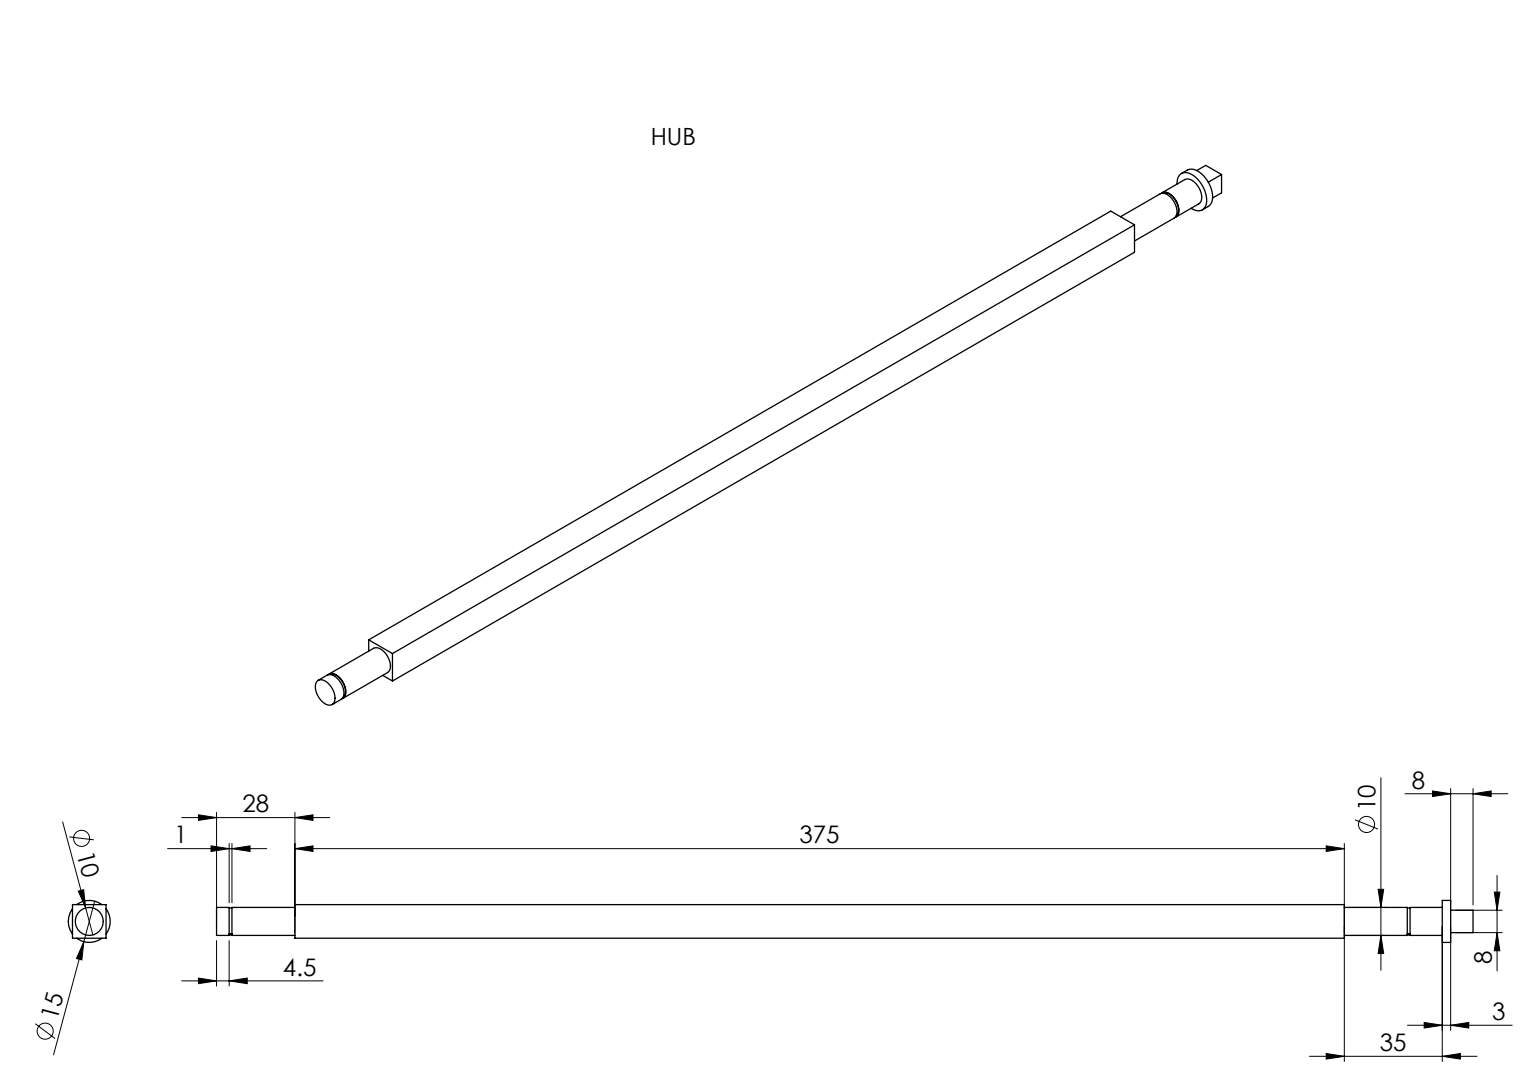
ISO-10303-21;
HEADER;
FILE_DESCRIPTION (('STEP AP214'),
    '1' );
FILE_NAME ('hub.step',
    '2026-10-27T17:01:19',
    ( '' ),
    ( '' ),
    'SwSTEP 2.0',
    'SolidWorks 2026',
    '' );
FILE_SCHEMA (( 'AUTOMOTIVE_DESIGN' ));
ENDSEC;

DATA;
#11=FACE_OUTER_BOUND ( 'NONE', #11887, .T. ) ;
#14=CARTESIAN_POINT ( 'NONE',  ( 640.0000000000000000, 160.0000000000000284, -222.5000000000000000 ) ) ;
#23=ORIENTED_EDGE ( 'NONE', *, *, #607, .T. ) ;
#30=VERTEX_POINT ( 'NONE', #596 ) ;
#33=ORIENTED_EDGE ( 'NONE', *, *, #12524, .T. ) ;
#37=CARTESIAN_POINT ( 'NONE',  ( 0.000000000000000000, 0.000000000000000000, -187.5000000000000000 ) ) ;
#38=ADVANCED_FACE ( 'NONE', ( #6155 ), #1724, .F. ) ;
#53=CARTESIAN_POINT ( 'NONE',  ( 629.0000000000000000, 166.0000000000000284, -187.5000000000000000 ) ) ;
#55=EDGE_LOOP ( 'NONE', ( #10980, #1481, #10748, #12698 ) ) ;
#70=PLANE ( 'NONE',  #7516 ) ;
#99=EDGE_LOOP ( 'NONE', ( #7071, #6114, #7487, #2779 ) ) ;
#101=DIRECTION ( 'NONE',  ( 0.000000000000000000, 0.000000000000000000, 1.000000000000000000 ) ) ;
#128=CARTESIAN_POINT ( 'NONE',  ( 630.0000000000000000, 160.0000000000000284, 215.5000000000000000 ) ) ;
#138=DIRECTION ( 'NONE',  ( -1.000000000000000000, 0.000000000000000000, 0.000000000000000000 ) ) ;
#142=CIRCLE ( 'NONE', #4214, 5.000000000000004441 ) ;
#146=DIRECTION ( 'NONE',  ( 0.000000000000000000, 0.000000000000000000, -1.000000000000000000 ) ) ;
#171=ORIENTED_EDGE ( 'NONE', *, *, #13700, .T. ) ;
#178=DIRECTION ( 'NONE',  ( 0.000000000000000000, 0.000000000000000000, -1.000000000000000000 ) ) ;
#203=AXIS2_PLACEMENT_3D ( 'NONE', #4127, #790, #8616 ) ;
#206=ADVANCED_FACE ( 'NONE', ( #6452 ), #11002, .F. ) ;
#207=ORIENTED_EDGE ( 'NONE', *, *, #12524, .F. ) ;
#218=EDGE_CURVE ( 'NONE', #4236, #7201, #9506, .T. ) ;
#230=DIRECTION ( 'NONE',  ( -1.000000000000000000, 0.000000000000000000, 0.000000000000000000 ) ) ;
#231=CARTESIAN_POINT ( 'NONE',  ( 635.0000000000000000, 160.0000000000000284, 215.5000000000000000 ) ) ;
#247=LINE ( 'NONE', #13705, #494 ) ;
#255=ORIENTED_EDGE ( 'NONE', *, *, #504, .F. ) ;
#267=CARTESIAN_POINT ( 'NONE',  ( 635.0000000000000000, 160.0000000000000284, 211.0000000000000000 ) ) ;
#274=ORIENTED_EDGE ( 'NONE', *, *, #3153, .F. ) ;
#302=EDGE_CURVE ( 'NONE', #2242, #4648, #7848, .T. ) ;
#309=EDGE_LOOP ( 'NONE', ( #11418, #2643 ) ) ;
#331=LINE ( 'NONE', #7064, #10396 ) ;
#344=VERTEX_POINT ( 'NONE', #128 ) ;
#361=DIRECTION ( 'NONE',  ( -1.000000000000000000, 0.000000000000000000, 0.000000000000000000 ) ) ;
#375=CARTESIAN_POINT ( 'NONE',  ( 637.0568832135862749, 155.4426727739092655, 210.0000000000000000 ) ) ;
#382=VECTOR ( 'NONE', #10428, 1000.000000000000000 ) ;
#383=DIRECTION ( 'NONE',  ( -2.312964634635740689E-15, 1.000000000000000000, 0.000000000000000000 ) ) ;
#390=( LENGTH_UNIT ( ) NAMED_UNIT ( * ) SI_UNIT ( .MILLI., .METRE. ) );
#403=EDGE_CURVE ( 'NONE', #12048, #8669, #5831, .T. ) ;
#426=EDGE_CURVE ( 'NONE', #4433, #3772, #8407, .T. ) ;
#433=VECTOR ( 'NONE', #6248, 1000.000000000000114 ) ;
#443=VERTEX_POINT ( 'NONE', #11657 ) ;
#471=CARTESIAN_POINT ( 'NONE',  ( 635.0000000000000000, 160.0000000000000284, -210.0000000000000000 ) ) ;
#482=( NAMED_UNIT ( * ) SI_UNIT ( $, .STERADIAN. ) SOLID_ANGLE_UNIT ( ) );
#491=VECTOR ( 'NONE', #11619, 1000.000000000000000 ) ;
#492=DIRECTION ( 'NONE',  ( 0.000000000000000000, 1.000000000000000000, 0.000000000000000000 ) ) ;
#494=VECTOR ( 'NONE', #2319, 1000.000000000000000 ) ;
#504=EDGE_CURVE ( 'NONE', #30, #10347, #1051, .T. ) ;
#509=ORIENTED_EDGE ( 'NONE', *, *, #9465, .F. ) ;
#512=VECTOR ( 'NONE', #1432, 1000.000000000000000 ) ;
#514=LINE ( 'NONE', #1705, #2365 ) ;
#515=PRODUCT_DEFINITION_FORMATION_WITH_SPECIFIED_SOURCE ( 'ANY', '', #13038, .NOT_KNOWN. ) ;
#531=EDGE_LOOP ( 'NONE', ( #7577, #12820, #549, #541 ) ) ;
#541=ORIENTED_EDGE ( 'NONE', *, *, #5828, .T. ) ;
#549=ORIENTED_EDGE ( 'NONE', *, *, #9465, .T. ) ;
#579=DIRECTION ( 'NONE',  ( -0.4113766427172328433, 0.9114654452181377708, 0.000000000000000000 ) ) ;
#587=LINE ( 'NONE', #6359, #4201 ) ;
#596=CARTESIAN_POINT ( 'NONE',  ( 630.5661054975340676, 158.1613647612965110, -210.0000000000000000 ) ) ;
#602=ORIENTED_EDGE ( 'NONE', *, *, #7925, .T. ) ;
#607=EDGE_CURVE ( 'NONE', #443, #1513, #6269, .T. ) ;
#623=AXIS2_PLACEMENT_3D ( 'NONE', #7389, #649, #7452 ) ;
#649=DIRECTION ( 'NONE',  ( 0.000000000000000000, 0.000000000000000000, 1.000000000000000000 ) ) ;
#659=DIRECTION ( 'NONE',  ( 0.9351104457158685435, 0.3543563944859322579, 0.000000000000000000 ) ) ;
#669=PLANE ( 'NONE',  #940 ) ;
#677=EDGE_CURVE ( 'NONE', #8007, #9101, #13359, .T. ) ;
#682=CARTESIAN_POINT ( 'NONE',  ( 636.7009106935324780, 155.5114698605638637, 210.0000000000000000 ) ) ;
#687=ORIENTED_EDGE ( 'NONE', *, *, #8817, .F. ) ;
#707=PLANE ( 'NONE',  #10370 ) ;
#708=VECTOR ( 'NONE', #14194, 1000.000000000000000 ) ;
#716=DIRECTION ( 'NONE',  ( 0.000000000000000000, 0.000000000000000000, -1.000000000000000000 ) ) ;
#724=ORIENTED_EDGE ( 'NONE', *, *, #11799, .T. ) ;
#728=CARTESIAN_POINT ( 'NONE',  ( 639.4338945024659324, 161.8386352387035743, 211.0000000000000000 ) ) ;
#730=DIRECTION ( 'NONE',  ( 1.000000000000000000, 0.000000000000000000, 0.000000000000000000 ) ) ;
#745=ADVANCED_FACE ( 'NONE', ( #7680 ), #12162, .T. ) ;
#771=DIRECTION ( 'NONE',  ( 1.000000000000000000, 0.000000000000000000, 0.000000000000000000 ) ) ;
#778=DIRECTION ( 'NONE',  ( -0.9237280213470676626, -0.3830490080632388272, 0.000000000000000000 ) ) ;
#790=DIRECTION ( 'NONE',  ( -0.000000000000000000, -0.000000000000000000, -1.000000000000000000 ) ) ;
#792=CARTESIAN_POINT ( 'NONE',  ( 640.0000000000000000, 160.0000000000000284, 211.0000000000000000 ) ) ;
#838=DIRECTION ( 'NONE',  ( -0.000000000000000000, -0.000000000000000000, 1.000000000000000000 ) ) ;
#865=LINE ( 'NONE', #5382, #12271 ) ;
#867=ORIENTED_EDGE ( 'NONE', *, *, #10385, .F. ) ;
#894=ORIENTED_EDGE ( 'NONE', *, *, #607, .F. ) ;
#904=CARTESIAN_POINT ( 'NONE',  ( 632.5000000000001137, 160.0000000000000284, -233.5000000000000000 ) ) ;
#905=LINE ( 'NONE', #5430, #12478 ) ;
#909=CARTESIAN_POINT ( 'NONE',  ( 631.0000000000000000, 155.9999999999999432, -225.5000000000000000 ) ) ;
#917=ORIENTED_EDGE ( 'NONE', *, *, #4871, .F. ) ;
#936=VECTOR ( 'NONE', #1493, 1000.000000000000000 ) ;
#940=AXIS2_PLACEMENT_3D ( 'NONE', #8922, #13348, #12233 ) ;
#984=ORIENTED_EDGE ( 'NONE', *, *, #2925, .F. ) ;
#991=PLANE ( 'NONE',  #8794 ) ;
#1042=ORIENTED_EDGE ( 'NONE', *, *, #13602, .T. ) ;
#1045=CARTESIAN_POINT ( 'NONE',  ( 635.0000000000000000, 160.0000000000000284, 215.5000000000000000 ) ) ;
#1048=EDGE_CURVE ( 'NONE', #344, #12114, #2171, .T. ) ;
#1051=CIRCLE ( 'NONE', #11204, 4.799999999999968736 ) ;
#1063=EDGE_LOOP ( 'NONE', ( #6144, #5179, #8194, #1305 ) ) ;
#1071=VERTEX_POINT ( 'NONE', #4391 ) ;
#1075=DIRECTION ( 'NONE',  ( 0.000000000000000000, 0.000000000000000000, -1.000000000000000000 ) ) ;
#1079=EDGE_CURVE ( 'NONE', #7687, #12048, #11107, .T. ) ;
#1090=ORIENTED_EDGE ( 'NONE', *, *, #6198, .F. ) ;
#1106=VECTOR ( 'NONE', #4618, 1000.000000000000000 ) ;
#1112=ORIENTED_EDGE ( 'NONE', *, *, #14048, .T. ) ;
#1114=DIRECTION ( 'NONE',  ( -0.4113766427172328433, 0.9114654452181377708, 0.000000000000000000 ) ) ;
#1119=EDGE_CURVE ( 'NONE', #14292, #9101, #13687, .T. ) ;
#1164=AXIS2_PLACEMENT_3D ( 'NONE', #12417, #11320, #11395 ) ;
#1184=AXIS2_PLACEMENT_3D ( 'NONE', #4149, #6216, #4000 ) ;
#1186=ORIENTED_EDGE ( 'NONE', *, *, #302, .F. ) ;
#1196=AXIS2_PLACEMENT_3D ( 'NONE', #8787, #1988, #730 ) ;
#1252=DIRECTION ( 'NONE',  ( -1.000000000000000000, 0.000000000000000000, 0.000000000000000000 ) ) ;
#1278=CYLINDRICAL_SURFACE ( 'NONE', #2591, 5.000000000000004441 ) ;
#1295=EDGE_CURVE ( 'NONE', #10237, #8326, #1789, .T. ) ;
#1305=ORIENTED_EDGE ( 'NONE', *, *, #9512, .F. ) ;
#1312=EDGE_CURVE ( 'NONE', #9111, #7367, #10328, .T. ) ;
#1328=ORIENTED_EDGE ( 'NONE', *, *, #14247, .F. ) ;
#1343=CARTESIAN_POINT ( 'NONE',  ( 635.0000000000000000, 160.0000000000000284, 210.0000000000000000 ) ) ;
#1353=CYLINDRICAL_SURFACE ( 'NONE', #2567, 4.799999999999968736 ) ;
#1363=PLANE ( 'NONE',  #4282 ) ;
#1388=AXIS2_PLACEMENT_3D ( 'NONE', #11311, #6806, #2160 ) ;
#1389=AXIS2_PLACEMENT_3D ( 'NONE', #10788, #8284, #2823 ) ;
#1399=ORIENTED_EDGE ( 'NONE', *, *, #2767, .F. ) ;
#1415=CARTESIAN_POINT ( 'NONE',  ( 639.0000000000000000, 156.0000000000000000, -233.5000000000000000 ) ) ;
#1429=VECTOR ( 'NONE', #9770, 1000.000000000000000 ) ;
#1431=EDGE_LOOP ( 'NONE', ( #8093, #11408, #3433, #2468 ) ) ;
#1432=DIRECTION ( 'NONE',  ( 0.000000000000000000, -1.000000000000000000, 0.000000000000000000 ) ) ;
#1450=EDGE_LOOP ( 'NONE', ( #12786, #4351, #13329, #7081 ) ) ;
#1467=DIRECTION ( 'NONE',  ( -0.4113766427172327877, 0.9114654452181378819, 0.000000000000000000 ) ) ;
#1469=ORIENTED_EDGE ( 'NONE', *, *, #13140, .F. ) ;
#1471=EDGE_CURVE ( 'NONE', #8142, #6053, #12201, .T. ) ;
#1481=ORIENTED_EDGE ( 'NONE', *, *, #4412, .T. ) ;
#1493=DIRECTION ( 'NONE',  ( -0.000000000000000000, -1.000000000000000000, -0.000000000000000000 ) ) ;
#1508=APPLICATION_CONTEXT ( 'automotive_design' ) ;
#1513=VERTEX_POINT ( 'NONE', #10945 ) ;
#1556=ORIENTED_EDGE ( 'NONE', *, *, #3833, .F. ) ;
#1581=LINE ( 'NONE', #6240, #6770 ) ;
#1597=AXIS2_PLACEMENT_3D ( 'NONE', #8501, #1930, #12858 ) ;
#1602=EDGE_CURVE ( 'NONE', #9849, #7148, #142, .T. ) ;
#1604=CYLINDRICAL_SURFACE ( 'NONE', #12074, 2.499999999999946709 ) ;
#1613=VECTOR ( 'NONE', #7698, 1000.000000000000227 ) ;
#1621=CIRCLE ( 'NONE', #4452, 7.500000000000062172 ) ;
#1645=AXIS2_PLACEMENT_3D ( 'NONE', #13635, #178, #7063 ) ;
#1656=CIRCLE ( 'NONE', #9902, 5.000000000000004441 ) ;
#1705=CARTESIAN_POINT ( 'NONE',  ( 640.0000000000000000, 160.0000000000000284, -222.5000000000000000 ) ) ;
#1717=FACE_OUTER_BOUND ( 'NONE', #6938, .T. ) ;
#1720=CIRCLE ( 'NONE', #13740, 5.000000000000004441 ) ;
#1721=CYLINDRICAL_SURFACE ( 'NONE', #1389, 5.000000000000004441 ) ;
#1724=PLANE ( 'NONE',  #5734 ) ;
#1764=DIRECTION ( 'NONE',  ( -0.000000000000000000, -0.000000000000000000, 1.000000000000000000 ) ) ;
#1773=DIRECTION ( 'NONE',  ( -0.9237280213470676626, -0.3830490080632388272, 0.000000000000000000 ) ) ;
#1774=ORIENTED_EDGE ( 'NONE', *, *, #9647, .T. ) ;
#1789=LINE ( 'NONE', #2689, #13155 ) ;
#1831=VECTOR ( 'NONE', #3586, 1000.000000000000000 ) ;
#1867=CIRCLE ( 'NONE', #6348, 5.000000000000004441 ) ;
#1881=CARTESIAN_POINT ( 'NONE',  ( 635.0000000000000000, 160.0000000000000284, 187.5000000000000000 ) ) ;
#1885=AXIS2_PLACEMENT_3D ( 'NONE', #11601, #12788, #8198 ) ;
#1911=VECTOR ( 'NONE', #7042, 1000.000000000000227 ) ;
#1919=CARTESIAN_POINT ( 'NONE',  ( 636.7009106935324780, 155.5114698605638637, -210.0000000000000000 ) ) ;
#1929=AXIS2_PLACEMENT_3D ( 'NONE', #1881, #9719, #771 ) ;
#1930=DIRECTION ( 'NONE',  ( 0.000000000000000000, 0.000000000000000000, -1.000000000000000000 ) ) ;
#1938=AXIS2_PLACEMENT_3D ( 'NONE', #9662, #6257, #4942 ) ;
#1944=DIRECTION ( 'NONE',  ( 0.000000000000000000, 0.000000000000000000, -1.000000000000000000 ) ) ;
#1988=DIRECTION ( 'NONE',  ( 0.000000000000000000, 0.000000000000000000, 1.000000000000000000 ) ) ;
#1990=EDGE_LOOP ( 'NONE', ( #5741, #984, #8590, #6479, #10508, #8888, #12809, #6092 ) ) ;
#1999=ORIENTED_EDGE ( 'NONE', *, *, #2925, .T. ) ;
#2010=CARTESIAN_POINT ( 'NONE',  ( 639.4338945024659324, 161.8386352387035743, -211.0000000000000000 ) ) ;
#2021=EDGE_CURVE ( 'NONE', #5281, #4527, #10031, .T. ) ;
#2025=CARTESIAN_POINT ( 'NONE',  ( 636.9746078850427011, 155.6249658629529620, 211.0000000000000000 ) ) ;
#2033=CARTESIAN_POINT ( 'NONE',  ( 631.0000000000000000, 164.0000000000000284, -225.5000000000000000 ) ) ;
#2054=AXIS2_PLACEMENT_3D ( 'NONE', #5135, #11687, #9343 ) ;
#2071=DIRECTION ( 'NONE',  ( 1.000000000000000000, 0.000000000000000000, 0.000000000000000000 ) ) ;
#2077=CIRCLE ( 'NONE', #5386, 5.000000000000004441 ) ;
#2079=CARTESIAN_POINT ( 'NONE',  ( 636.9746078850427011, 155.6249658629529620, 211.0000000000000000 ) ) ;
#2095=ORIENTED_EDGE ( 'NONE', *, *, #11278, .T. ) ;
#2124=DIRECTION ( 'NONE',  ( 0.000000000000000000, 0.000000000000000000, -1.000000000000000000 ) ) ;
#2151=EDGE_CURVE ( 'NONE', #5281, #6413, #9447, .T. ) ;
#2155=LINE ( 'NONE', #12566, #8727 ) ;
#2160=DIRECTION ( 'NONE',  ( -1.000000000000000000, 0.000000000000000000, 0.000000000000000000 ) ) ;
#2171=LINE ( 'NONE', #6533, #3024 ) ;
#2186=EDGE_LOOP ( 'NONE', ( #11729, #3232, #3231, #11948, #2256, #7091, #1090, #687 ) ) ;
#2210=ORIENTED_EDGE ( 'NONE', *, *, #2498, .T. ) ;
#2223=DIRECTION ( 'NONE',  ( -0.000000000000000000, -0.000000000000000000, 1.000000000000000000 ) ) ;
#2227=CARTESIAN_POINT ( 'NONE',  ( 637.5000000000000000, 160.0000000000000284, -217.5000000000000284 ) ) ;
#2242=VERTEX_POINT ( 'NONE', #9805 ) ;
#2244=ORIENTED_EDGE ( 'NONE', *, *, #504, .T. ) ;
#2251=DIRECTION ( 'NONE',  ( -0.4113766427172327877, 0.9114654452181378819, 0.000000000000000000 ) ) ;
#2256=ORIENTED_EDGE ( 'NONE', *, *, #2297, .F. ) ;
#2272=AXIS2_PLACEMENT_3D ( 'NONE', #11062, #14534, #11281 ) ;
#2278=CIRCLE ( 'NONE', #10307, 5.000000000000004441 ) ;
#2281=LINE ( 'NONE', #8788, #13228 ) ;
#2285=AXIS2_PLACEMENT_3D ( 'NONE', #2392, #8964, #7790 ) ;
#2289=PLANE ( 'NONE',  #4257 ) ;
#2293=FACE_OUTER_BOUND ( 'NONE', #7234, .T. ) ;
#2297=EDGE_CURVE ( 'NONE', #4638, #8007, #1581, .T. ) ;
#2298=VERTEX_POINT ( 'NONE', #2700 ) ;
#2303=CYLINDRICAL_SURFACE ( 'NONE', #2285, 2.499999999999946709 ) ;
#2313=ORIENTED_EDGE ( 'NONE', *, *, #13602, .F. ) ;
#2315=CARTESIAN_POINT ( 'NONE',  ( 632.5000000000001137, 160.0000000000000284, -233.5000000000000000 ) ) ;
#2316=ADVANCED_FACE ( 'NONE', ( #2634 ), #7200, .T. ) ;
#2319=DIRECTION ( 'NONE',  ( 1.000000000000000000, -3.469446951953611033E-15, -0.000000000000000000 ) ) ;
#2336=ADVANCED_FACE ( 'NONE', ( #8304 ), #4032, .F. ) ;
#2358=VERTEX_POINT ( 'NONE', #14005 ) ;
#2360=DIRECTION ( 'NONE',  ( 1.000000000000000000, 0.000000000000000000, 0.000000000000000000 ) ) ;
#2362=CIRCLE ( 'NONE', #10864, 5.000000000000004441 ) ;
#2365=VECTOR ( 'NONE', #1764, 1000.000000000000000 ) ;
#2370=AXIS2_PLACEMENT_3D ( 'NONE', #13791, #11566, #1467 ) ;
#2372=CARTESIAN_POINT ( 'NONE',  ( 635.0000000000000000, 160.0000000000000284, 211.0000000000000000 ) ) ;
#2392=CARTESIAN_POINT ( 'NONE',  ( 635.0000000000000000, 160.0000000000000284, -233.5000000000000000 ) ) ;
#2400=LINE ( 'NONE', #2315, #10872 ) ;
#2403=AXIS2_PLACEMENT_3D ( 'NONE', #10500, #5059, #10437 ) ;
#2431=CYLINDRICAL_SURFACE ( 'NONE', #7085, 4.799999999999968736 ) ;
#2443=DIRECTION ( 'NONE',  ( -0.000000000000000000, -0.000000000000000000, 1.000000000000000000 ) ) ;
#2448=DIRECTION ( 'NONE',  ( -0.9237280213470676626, -0.3830490080632388272, 0.000000000000000000 ) ) ;
#2450=DIRECTION ( 'NONE',  ( 0.3543563944859323134, -0.9351104457158685435, 0.000000000000000000 ) ) ;
#2464=DIRECTION ( 'NONE',  ( -1.000000000000000000, 0.000000000000000000, 0.000000000000000000 ) ) ;
#2468=ORIENTED_EDGE ( 'NONE', *, *, #13088, .F. ) ;
#2472=ORIENTED_EDGE ( 'NONE', *, *, #13700, .F. ) ;
#2474=EDGE_CURVE ( 'NONE', #9849, #7201, #587, .T. ) ;
#2481=ADVANCED_FACE ( 'NONE', ( #1717 ), #6220, .F. ) ;
#2483=CARTESIAN_POINT ( 'NONE',  ( 635.0000000000000000, 160.0000000000000284, -225.5000000000000000 ) ) ;
#2491=PLANE ( 'NONE',  #13452 ) ;
#2496=LINE ( 'NONE', #8384, #433 ) ;
#2498=EDGE_CURVE ( 'NONE', #12112, #1071, #5144, .T. ) ;
#2512=LINE ( 'NONE', #1415, #936 ) ;
#2532=DIRECTION ( 'NONE',  ( -1.000000000000000000, 0.000000000000000000, 0.000000000000000000 ) ) ;
#2542=CARTESIAN_POINT ( 'NONE',  ( 637.0568832135862749, 155.4426727739092655, -211.0000000000000000 ) ) ;
#2557=MANIFOLD_SOLID_BREP ( 'AdvancedHole1', #11148 ) ;
#2567=AXIS2_PLACEMENT_3D ( 'NONE', #4312, #9774, #8513 ) ;
#2579=ORIENTED_EDGE ( 'NONE', *, *, #2767, .T. ) ;
#2583=CARTESIAN_POINT ( 'NONE',  ( 639.0000000000000000, 156.0000000000000000, -233.5000000000000000 ) ) ;
#2591=AXIS2_PLACEMENT_3D ( 'NONE', #1045, #5843, #138 ) ;
#2625=ORIENTED_EDGE ( 'NONE', *, *, #6511, .T. ) ;
#2628=VECTOR ( 'NONE', #8665, 1000.000000000000000 ) ;
#2634=FACE_OUTER_BOUND ( 'NONE', #5663, .T. ) ;
#2643=ORIENTED_EDGE ( 'NONE', *, *, #12581, .F. ) ;
#2650=PLANE ( 'NONE',  #6633 ) ;
#2656=EDGE_LOOP ( 'NONE', ( #724, #9745, #8062, #171, #7414, #5546, #2244, #3375 ) ) ;
#2689=CARTESIAN_POINT ( 'NONE',  ( 641.0000000000000000, 166.0000000000000284, -187.5000000000000000 ) ) ;
#2700=CARTESIAN_POINT ( 'NONE',  ( 640.0000000000000000, 160.0000000000000284, -211.0000000000000000 ) ) ;
#2720=CARTESIAN_POINT ( 'NONE',  ( 631.0000000000000000, 155.9999999999999432, -233.5000000000000000 ) ) ;
#2721=VERTEX_POINT ( 'NONE', #8479 ) ;
#2732=VERTEX_POINT ( 'NONE', #8400 ) ;
#2767=EDGE_CURVE ( 'NONE', #9543, #11816, #14246, .T. ) ;
#2773=SHAPE_REPRESENTATION_RELATIONSHIP ( 'NONE' , 'NONE' ,  #9980, #6513 ) ;
#2779=ORIENTED_EDGE ( 'NONE', *, *, #10399, .F. ) ;
#2786=EDGE_CURVE ( 'NONE', #6408, #4046, #2077, .T. ) ;
#2787=DIRECTION ( 'NONE',  ( -0.000000000000000000, -0.000000000000000000, -1.000000000000000000 ) ) ;
#2795=CIRCLE ( 'NONE', #11039, 4.799999999999968736 ) ;
#2815=EDGE_LOOP ( 'NONE', ( #274, #13787, #14344, #12061 ) ) ;
#2823=DIRECTION ( 'NONE',  ( -1.000000000000000000, 0.000000000000000000, 0.000000000000000000 ) ) ;
#2843=PLANE ( 'NONE',  #8956 ) ;
#2853=SURFACE_STYLE_FILL_AREA ( #8232 ) ;
#2867=DIRECTION ( 'NONE',  ( 0.000000000000000000, 0.000000000000000000, -1.000000000000000000 ) ) ;
#2871=DIRECTION ( 'NONE',  ( -0.000000000000000000, 0.000000000000000000, -1.000000000000000000 ) ) ;
#2884=ADVANCED_FACE ( 'NONE', ( #14603 ), #10924, .T. ) ;
#2896=DIRECTION ( 'NONE',  ( -1.000000000000000000, 0.000000000000000000, 0.000000000000000000 ) ) ;
#2900=VECTOR ( 'NONE', #3639, 1000.000000000000000 ) ;
#2909=ORIENTED_EDGE ( 'NONE', *, *, #10247, .F. ) ;
#2915=CARTESIAN_POINT ( 'NONE',  ( 637.5000000000000000, 160.0000000000000284, -217.5000000000000284 ) ) ;
#2925=EDGE_CURVE ( 'NONE', #11833, #9079, #2795, .T. ) ;
#2935=ORIENTED_EDGE ( 'NONE', *, *, #1079, .T. ) ;
#2937=ADVANCED_FACE ( 'NONE', ( #9212, #12600 ), #10466, .F. ) ;
#2945=ADVANCED_FACE ( 'NONE', ( #4864, #4573 ), #13854, .T. ) ;
#2995=ORIENTED_EDGE ( 'NONE', *, *, #8081, .T. ) ;
#3007=ORIENTED_EDGE ( 'NONE', *, *, #2021, .F. ) ;
#3024=VECTOR ( 'NONE', #12983, 1000.000000000000000 ) ;
#3043=CONICAL_SURFACE ( 'NONE', #1388, 2.499999999999946709, 1.029744259999984646 ) ;
#3045=CIRCLE ( 'NONE', #10351, 5.000000000000004441 ) ;
#3060=CARTESIAN_POINT ( 'NONE',  ( 640.0000000000000000, 160.0000000000000284, -210.0000000000000000 ) ) ;
#3063=CARTESIAN_POINT ( 'NONE',  ( 630.5661054975340676, 158.1613647612965110, -210.0000000000000000 ) ) ;
#3120=LINE ( 'NONE', #5398, #9676 ) ;
#3134=ORIENTED_EDGE ( 'NONE', *, *, #6198, .T. ) ;
#3142=AXIS2_PLACEMENT_3D ( 'NONE', #6667, #12255, #11160 ) ;
#3153=EDGE_CURVE ( 'NONE', #3214, #9710, #12894, .T. ) ;
#3177=ADVANCED_FACE ( 'NONE', ( #8818 ), #70, .F. ) ;
#3202=DIRECTION ( 'NONE',  ( -0.000000000000000000, -0.000000000000000000, -1.000000000000000000 ) ) ;
#3214=VERTEX_POINT ( 'NONE', #2227 ) ;
#3226=EDGE_CURVE ( 'NONE', #6053, #8142, #1621, .T. ) ;
#3230=CARTESIAN_POINT ( 'NONE',  ( 640.0000000000000000, 160.0000000000000284, 210.0000000000000000 ) ) ;
#3231=ORIENTED_EDGE ( 'NONE', *, *, #9010, .F. ) ;
#3232=ORIENTED_EDGE ( 'NONE', *, *, #9647, .F. ) ;
#3235=ADVANCED_FACE ( 'NONE', ( #2293 ), #3043, .F. ) ;
#3241=CARTESIAN_POINT ( 'NONE',  ( 629.0000000000000000, 166.0000000000000284, 187.5000000000000000 ) ) ;
#3243=ORIENTED_EDGE ( 'NONE', *, *, #2297, .T. ) ;
#3250=AXIS2_PLACEMENT_3D ( 'NONE', #3727, #230, #3809 ) ;
#3259=VECTOR ( 'NONE', #13471, 1000.000000000000000 ) ;
#3264=DIRECTION ( 'NONE',  ( -0.000000000000000000, -0.000000000000000000, -1.000000000000000000 ) ) ;
#3268=DIRECTION ( 'NONE',  ( 0.000000000000000000, 0.000000000000000000, 1.000000000000000000 ) ) ;
#3366=FACE_OUTER_BOUND ( 'NONE', #5624, .T. ) ;
#3375=ORIENTED_EDGE ( 'NONE', *, *, #13140, .T. ) ;
#3387=CARTESIAN_POINT ( 'NONE',  ( 635.0000000000000000, 160.0000000000000284, -215.9978484569338946 ) ) ;
#3416=CARTESIAN_POINT ( 'NONE',  ( 639.0000000000000000, 156.0000000000000000, -225.5000000000000000 ) ) ;
#3425=ORIENTED_EDGE ( 'NONE', *, *, #426, .F. ) ;
#3429=CARTESIAN_POINT ( 'NONE',  ( 641.0000000000000000, 166.0000000000000284, 187.5000000000000000 ) ) ;
#3433=ORIENTED_EDGE ( 'NONE', *, *, #8898, .F. ) ;
#3439=FACE_OUTER_BOUND ( 'NONE', #5993, .T. ) ;
#3466=ORIENTED_EDGE ( 'NONE', *, *, #13862, .F. ) ;
#3472=CARTESIAN_POINT ( 'NONE',  ( 639.0000000000000000, 164.0000000000000000, -233.5000000000000000 ) ) ;
#3480=ORIENTED_EDGE ( 'NONE', *, *, #7191, .T. ) ;
#3482=DIRECTION ( 'NONE',  ( -1.000000000000000000, 0.000000000000000000, 0.000000000000000000 ) ) ;
#3483=CARTESIAN_POINT ( 'NONE',  ( 635.0000000000000000, 160.0000000000000284, -233.5000000000000000 ) ) ;
#3509=CARTESIAN_POINT ( 'NONE',  ( 636.7009106935324780, 155.5114698605638637, 210.0000000000000000 ) ) ;
#3530=AXIS2_PLACEMENT_3D ( 'NONE', #4010, #12862, #4093 ) ;
#3537=CIRCLE ( 'NONE', #1645, 5.000000000000004441 ) ;
#3551=ORIENTED_EDGE ( 'NONE', *, *, #2786, .F. ) ;
#3554=AXIS2_PLACEMENT_3D ( 'NONE', #4646, #5813, #1252 ) ;
#3565=STYLED_ITEM ( 'NONE', ( #12743 ), #6513 ) ;
#3586=DIRECTION ( 'NONE',  ( 0.000000000000000000, 0.000000000000000000, -1.000000000000000000 ) ) ;
#3601=CARTESIAN_POINT ( 'NONE',  ( 635.0000000000000000, 160.0000000000000284, 210.0000000000000000 ) ) ;
#3612=DIRECTION ( 'NONE',  ( 0.000000000000000000, 0.000000000000000000, -1.000000000000000000 ) ) ;
#3615=DIRECTION ( 'NONE',  ( -0.9237280213470676626, -0.3830490080632388272, 0.000000000000000000 ) ) ;
#3617=FACE_OUTER_BOUND ( 'NONE', #5453, .T. ) ;
#3630=ORIENTED_EDGE ( 'NONE', *, *, #426, .T. ) ;
#3639=DIRECTION ( 'NONE',  ( -0.000000000000000000, -0.000000000000000000, 1.000000000000000000 ) ) ;
#3648=DIRECTION ( 'NONE',  ( 0.000000000000000000, 0.000000000000000000, 1.000000000000000000 ) ) ;
#3649=FACE_OUTER_BOUND ( 'NONE', #55, .T. ) ;
#3660=VERTEX_POINT ( 'NONE', #4521 ) ;
#3678=DIRECTION ( 'NONE',  ( -0.000000000000000000, 0.000000000000000000, 1.000000000000000000 ) ) ;
#3716=CARTESIAN_POINT ( 'NONE',  ( 642.5000000000001137, 160.0000000000000284, -222.5000000000000000 ) ) ;
#3717=CYLINDRICAL_SURFACE ( 'NONE', #1885, 7.500000000000062172 ) ;
#3727=CARTESIAN_POINT ( 'NONE',  ( 639.0000000000000000, 156.0000000000000000, -233.5000000000000000 ) ) ;
#3746=LINE ( 'NONE', #7273, #8893 ) ;
#3755=EDGE_CURVE ( 'NONE', #4197, #5281, #11375, .T. ) ;
#3756=FACE_OUTER_BOUND ( 'NONE', #10506, .T. ) ;
#3772=VERTEX_POINT ( 'NONE', #6943 ) ;
#3783=DIRECTION ( 'NONE',  ( -1.000000000000000000, 0.000000000000000000, 0.000000000000000000 ) ) ;
#3809=DIRECTION ( 'NONE',  ( 0.000000000000000000, 0.000000000000000000, 1.000000000000000000 ) ) ;
#3812=ORIENTED_EDGE ( 'NONE', *, *, #7191, .F. ) ;
#3833=EDGE_CURVE ( 'NONE', #4638, #7367, #12554, .T. ) ;
#3839=EDGE_LOOP ( 'NONE', ( #10057, #7560, #8717 ) ) ;
#3874=DIRECTION ( 'NONE',  ( -0.8571673013836776933, 0.000000000000000000, -0.5150380737757388472 ) ) ;
#3889=FACE_OUTER_BOUND ( 'NONE', #6270, .T. ) ;
#3897=ORIENTED_EDGE ( 'NONE', *, *, #6283, .T. ) ;
#3918=CARTESIAN_POINT ( 'NONE',  ( 636.7717819724297215, 155.3244477714206653, 210.0000000000000000 ) ) ;
#3934=ORIENTED_EDGE ( 'NONE', *, *, #4412, .F. ) ;
#3950=DIRECTION ( 'NONE',  ( -0.9237280213470676626, -0.3830490080632388272, 0.000000000000000000 ) ) ;
#3976=CARTESIAN_POINT ( 'NONE',  ( 631.0000000000000000, 155.9999999999999432, -225.5000000000000000 ) ) ;
#3992=AXIS2_PLACEMENT_3D ( 'NONE', #6474, #838, #14229 ) ;
#3994=CARTESIAN_POINT ( 'NONE',  ( 636.9746078850427011, 155.6249658629529620, 211.0000000000000000 ) ) ;
#4000=DIRECTION ( 'NONE',  ( -0.9237280213470676626, -0.3830490080632388272, 0.000000000000000000 ) ) ;
#4010=CARTESIAN_POINT ( 'NONE',  ( 635.0000000000000000, 160.0000000000000284, -222.5000000000000000 ) ) ;
#4012=VERTEX_POINT ( 'NONE', #5463 ) ;
#4032=PLANE ( 'NONE',  #8421 ) ;
#4046=VERTEX_POINT ( 'NONE', #13500 ) ;
#4047=EDGE_CURVE ( 'NONE', #1071, #8142, #12377, .T. ) ;
#4051=LINE ( 'NONE', #11918, #13669 ) ;
#4060=LINE ( 'NONE', #3976, #14199 ) ;
#4074=CARTESIAN_POINT ( 'NONE',  ( 630.0000000000000000, 160.0000000000000284, -222.5000000000000000 ) ) ;
#4093=DIRECTION ( 'NONE',  ( 1.000000000000000000, 0.000000000000000000, 0.000000000000000000 ) ) ;
#4099=ORIENTED_EDGE ( 'NONE', *, *, #3755, .T. ) ;
#4105=CARTESIAN_POINT ( 'NONE',  ( 639.4338945024659324, 161.8386352387035743, 211.0000000000000000 ) ) ;
#4123=CARTESIAN_POINT ( 'NONE',  ( 635.0000000000000000, 160.0000000000000284, -222.5000000000000000 ) ) ;
#4127=CARTESIAN_POINT ( 'NONE',  ( 635.0000000000000000, 160.0000000000000284, -217.5000000000000284 ) ) ;
#4137=EDGE_CURVE ( 'NONE', #4046, #6408, #3537, .T. ) ;
#4149=CARTESIAN_POINT ( 'NONE',  ( 635.0000000000000000, 160.0000000000000284, -210.0000000000000000 ) ) ;
#4169=CARTESIAN_POINT ( 'NONE',  ( 641.0000000000000000, 166.0000000000000284, 187.5000000000000000 ) ) ;
#4175=CARTESIAN_POINT ( 'NONE',  ( 630.0000000000000000, 160.0000000000000284, 211.0000000000000000 ) ) ;
#4192=VECTOR ( 'NONE', #7930, 1000.000000000000000 ) ;
#4197=VERTEX_POINT ( 'NONE', #12603 ) ;
#4200=EDGE_CURVE ( 'NONE', #13817, #443, #13856, .T. ) ;
#4201=VECTOR ( 'NONE', #5111, 1000.000000000000000 ) ;
#4210=ORIENTED_EDGE ( 'NONE', *, *, #6506, .F. ) ;
#4211=VECTOR ( 'NONE', #7603, 1000.000000000000000 ) ;
#4214=AXIS2_PLACEMENT_3D ( 'NONE', #9315, #12336, #3482 ) ;
#4228=EDGE_CURVE ( 'NONE', #443, #4433, #4051, .T. ) ;
#4236=VERTEX_POINT ( 'NONE', #4935 ) ;
#4250=DIRECTION ( 'NONE',  ( -0.000000000000000000, -0.000000000000000000, 1.000000000000000000 ) ) ;
#4253=DIRECTION ( 'NONE',  ( -0.9237280213470682178, -0.3830490080632377725, 0.000000000000000000 ) ) ;
#4255=CIRCLE ( 'NONE', #10855, 4.799999999999968736 ) ;
#4256=ORIENTED_EDGE ( 'NONE', *, *, #2498, .F. ) ;
#4257=AXIS2_PLACEMENT_3D ( 'NONE', #4674, #5553, #6801 ) ;
#4282=AXIS2_PLACEMENT_3D ( 'NONE', #9414, #383, #10373 ) ;
#4295=CARTESIAN_POINT ( 'NONE',  ( 635.0000000000000000, 160.0000000000000284, 211.0000000000000000 ) ) ;
#4299=( LENGTH_UNIT ( ) NAMED_UNIT ( * ) SI_UNIT ( .MILLI., .METRE. ) );
#4300=DIRECTION ( 'NONE',  ( 0.000000000000000000, 0.000000000000000000, -1.000000000000000000 ) ) ;
#4312=CARTESIAN_POINT ( 'NONE',  ( 635.0000000000000000, 160.0000000000000284, 211.0000000000000000 ) ) ;
#4342=ORIENTED_EDGE ( 'NONE', *, *, #8898, .T. ) ;
#4347=CARTESIAN_POINT ( 'NONE',  ( 0.000000000000000000, 0.000000000000000000, 0.000000000000000000 ) ) ;
#4349=ADVANCED_FACE ( 'NONE', ( #8461 ), #707, .F. ) ;
#4351=ORIENTED_EDGE ( 'NONE', *, *, #7821, .T. ) ;
#4353=CARTESIAN_POINT ( 'NONE',  ( 640.0000000000000000, 160.0000000000000284, 215.5000000000000000 ) ) ;
#4358=DIRECTION ( 'NONE',  ( 1.000000000000000000, -3.469446951953611033E-15, -0.000000000000000000 ) ) ;
#4377=DIRECTION ( 'NONE',  ( -1.000000000000000000, 0.000000000000000000, 0.000000000000000000 ) ) ;
#4379=ORIENTED_EDGE ( 'NONE', *, *, #4583, .T. ) ;
#4391=CARTESIAN_POINT ( 'NONE',  ( 627.5000000000000000, 160.0000000000000284, -225.5000000000000000 ) ) ;
#4398=DIRECTION ( 'NONE',  ( 0.000000000000000000, 0.000000000000000000, 1.000000000000000000 ) ) ;
#4410=CARTESIAN_POINT ( 'NONE',  ( 630.0000000000000000, 160.0000000000000284, -211.0000000000000000 ) ) ;
#4411=ORIENTED_EDGE ( 'NONE', *, *, #12861, .F. ) ;
#4412=EDGE_CURVE ( 'NONE', #7148, #4236, #12079, .T. ) ;
#4424=LINE ( 'NONE', #3241, #1429 ) ;
#4433=VERTEX_POINT ( 'NONE', #6754 ) ;
#4438=CARTESIAN_POINT ( 'NONE',  ( 630.0000000000000000, 160.0000000000000284, 210.0000000000000000 ) ) ;
#4445=CARTESIAN_POINT ( 'NONE',  ( 635.0000000000000000, 160.0000000000000284, -217.5000000000000284 ) ) ;
#4452=AXIS2_PLACEMENT_3D ( 'NONE', #12407, #13597, #5496 ) ;
#4463=DIRECTION ( 'NONE',  ( 0.000000000000000000, -1.000000000000000000, 0.000000000000000000 ) ) ;
#4496=CIRCLE ( 'NONE', #1184, 4.799999999999968736 ) ;
#4510=CIRCLE ( 'NONE', #12036, 5.000000000000004441 ) ;
#4519=( NAMED_UNIT ( * ) SI_UNIT ( $, .STERADIAN. ) SOLID_ANGLE_UNIT ( ) );
#4521=CARTESIAN_POINT ( 'NONE',  ( 639.0000000000000000, 164.0000000000000000, -225.5000000000000000 ) ) ;
#4527=VERTEX_POINT ( 'NONE', #12144 ) ;
#4535=EDGE_LOOP ( 'NONE', ( #7873, #11476, #8879, #14354 ) ) ;
#4548=PLANE ( 'NONE',  #3250 ) ;
#4573=FACE_OUTER_BOUND ( 'NONE', #7783, .T. ) ;
#4580=CARTESIAN_POINT ( 'NONE',  ( 639.0000000000000000, 164.0000000000000000, -233.5000000000000000 ) ) ;
#4583=EDGE_CURVE ( 'NONE', #8326, #11698, #10372, .T. ) ;
#4584=DIRECTION ( 'NONE',  ( -0.000000000000000000, 0.000000000000000000, -1.000000000000000000 ) ) ;
#4588=ORIENTED_EDGE ( 'NONE', *, *, #5783, .T. ) ;
#4606=CARTESIAN_POINT ( 'NONE',  ( 636.9746078850427011, 155.6249658629529620, 210.0000000000000000 ) ) ;
#4615=CARTESIAN_POINT ( 'NONE',  ( 635.0000000000000000, 160.0000000000000284, -225.5000000000000000 ) ) ;
#4618=DIRECTION ( 'NONE',  ( 0.000000000000000000, 0.000000000000000000, -1.000000000000000000 ) ) ;
#4624=ORIENTED_EDGE ( 'NONE', *, *, #9717, .T. ) ;
#4628=DIRECTION ( 'NONE',  ( 0.000000000000000000, 0.000000000000000000, 1.000000000000000000 ) ) ;
#4635=ORIENTED_EDGE ( 'NONE', *, *, #9010, .T. ) ;
#4638=VERTEX_POINT ( 'NONE', #2542 ) ;
#4646=CARTESIAN_POINT ( 'NONE',  ( 635.0000000000000000, 160.0000000000000284, -211.0000000000000000 ) ) ;
#4648=VERTEX_POINT ( 'NONE', #9116 ) ;
#4657=EDGE_LOOP ( 'NONE', ( #12040, #4624 ) ) ;
#4660=CARTESIAN_POINT ( 'NONE',  ( 635.0000000000000000, 160.0000000000000284, 215.5000000000000000 ) ) ;
#4662=CIRCLE ( 'NONE', #5361, 4.799999999999968736 ) ;
#4674=CARTESIAN_POINT ( 'NONE',  ( 0.000000000000000000, 0.000000000000000000, -233.5000000000000000 ) ) ;
#4677=LINE ( 'NONE', #7022, #382 ) ;
#4709=DIRECTION ( 'NONE',  ( -1.000000000000000000, 0.000000000000000000, 0.000000000000000000 ) ) ;
#4717=VECTOR ( 'NONE', #13742, 1000.000000000000000 ) ;
#4718=ADVANCED_FACE ( 'NONE', ( #9565 ), #2843, .F. ) ;
#4734=FACE_OUTER_BOUND ( 'NONE', #1990, .T. ) ;
#4742=EDGE_LOOP ( 'NONE', ( #6867, #12768, #6697, #10922, #11115, #6041, #12911, #3480, #1186, #14101, #12099, #6702 ) ) ;
#4745=AXIS2_PLACEMENT_3D ( 'NONE', #471, #5071, #3950 ) ;
#4761=ORIENTED_EDGE ( 'NONE', *, *, #2474, .T. ) ;
#4777=ORIENTED_EDGE ( 'NONE', *, *, #1295, .T. ) ;
#4795=ADVANCED_FACE ( 'NONE', ( #3889 ), #7343, .T. ) ;
#4808=DIRECTION ( 'NONE',  ( 0.000000000000000000, 0.000000000000000000, -1.000000000000000000 ) ) ;
#4830=FACE_OUTER_BOUND ( 'NONE', #7515, .T. ) ;
#4833=EDGE_LOOP ( 'NONE', ( #12191, #3897, #5199, #9320 ) ) ;
#4864=FACE_BOUND ( 'NONE', #99, .T. ) ;
#4867=PLANE ( 'NONE',  #2370 ) ;
#4871=EDGE_CURVE ( 'NONE', #4433, #10237, #10890, .T. ) ;
#4907=EDGE_CURVE ( 'NONE', #30, #12192, #13171, .T. ) ;
#4910=FACE_OUTER_BOUND ( 'NONE', #1063, .T. ) ;
#4917=DIRECTION ( 'NONE',  ( -6.938893903907222067E-15, 1.000000000000000000, 0.000000000000000000 ) ) ;
#4926=AXIS2_PLACEMENT_3D ( 'NONE', #3483, #3264, #4377 ) ;
#4935=CARTESIAN_POINT ( 'NONE',  ( 640.0000000000000000, 160.0000000000000284, 187.5000000000000000 ) ) ;
#4936=DIRECTION ( 'NONE',  ( -0.000000000000000000, -0.000000000000000000, 1.000000000000000000 ) ) ;
#4942=DIRECTION ( 'NONE',  ( -1.000000000000000000, 0.000000000000000000, 0.000000000000000000 ) ) ;
#4957=CIRCLE ( 'NONE', #12951, 5.000000000000004441 ) ;
#4992=VECTOR ( 'NONE', #10479, 1000.000000000000000 ) ;
#5015=CIRCLE ( 'NONE', #1929, 5.000000000000004441 ) ;
#5027=ORIENTED_EDGE ( 'NONE', *, *, #4907, .F. ) ;
#5031=VERTEX_POINT ( 'NONE', #10214 ) ;
#5059=DIRECTION ( 'NONE',  ( 0.000000000000000000, 0.000000000000000000, -1.000000000000000000 ) ) ;
#5071=DIRECTION ( 'NONE',  ( 0.000000000000000000, 0.000000000000000000, -1.000000000000000000 ) ) ;
#5074=EDGE_LOOP ( 'NONE', ( #10981, #13032, #10388, #8298 ) ) ;
#5078=( NAMED_UNIT ( * ) SI_UNIT ( $, .STERADIAN. ) SOLID_ANGLE_UNIT ( ) );
#5080=CARTESIAN_POINT ( 'NONE',  ( 637.0568832135862749, 155.4426727739092655, -210.0000000000000000 ) ) ;
#5102=CARTESIAN_POINT ( 'NONE',  ( 635.0000000000000000, 160.0000000000000284, -210.0000000000000000 ) ) ;
#5111=DIRECTION ( 'NONE',  ( -0.000000000000000000, -0.000000000000000000, -1.000000000000000000 ) ) ;
#5123=CYLINDRICAL_SURFACE ( 'NONE', #13169, 7.500000000000062172 ) ;
#5128=VERTEX_POINT ( 'NONE', #728 ) ;
#5135=CARTESIAN_POINT ( 'NONE',  ( 635.0000000000000000, 160.0000000000000284, -210.0000000000000000 ) ) ;
#5144=CIRCLE ( 'NONE', #1597, 7.500000000000062172 ) ;
#5147=VERTEX_POINT ( 'NONE', #3918 ) ;
#5149=DIRECTION ( 'NONE',  ( 0.3543563944859323689, -0.9351104457158684324, 0.000000000000000000 ) ) ;
#5164=CONICAL_SURFACE ( 'NONE', #13403, 2.499999999999946709, 1.029744259999984646 ) ;
#5179=ORIENTED_EDGE ( 'NONE', *, *, #4047, .T. ) ;
#5182=DIRECTION ( 'NONE',  ( -0.9237280213470676626, -0.3830490080632388272, 0.000000000000000000 ) ) ;
#5199=ORIENTED_EDGE ( 'NONE', *, *, #8812, .T. ) ;
#5234=DIRECTION ( 'NONE',  ( 0.9351104457158685435, 0.3543563944859324244, 0.000000000000000000 ) ) ;
#5276=CARTESIAN_POINT ( 'NONE',  ( 635.0000000000000000, 160.0000000000000284, 211.0000000000000000 ) ) ;
#5281=VERTEX_POINT ( 'NONE', #8785 ) ;
#5301=ADVANCED_FACE ( 'NONE', ( #3617 ), #4867, .F. ) ;
#5313=DIRECTION ( 'NONE',  ( -1.000000000000000000, 0.000000000000000000, 0.000000000000000000 ) ) ;
#5347=EDGE_CURVE ( 'NONE', #4527, #13395, #331, .T. ) ;
#5357=CYLINDRICAL_SURFACE ( 'NONE', #3992, 5.000000000000004441 ) ;
#5361=AXIS2_PLACEMENT_3D ( 'NONE', #3601, #4628, #6975 ) ;
#5363=ADVANCED_FACE ( 'NONE', ( #3756 ), #11421, .T. ) ;
#5382=CARTESIAN_POINT ( 'NONE',  ( 639.0000000000000000, 164.0000000000000000, -225.5000000000000000 ) ) ;
#5386=AXIS2_PLACEMENT_3D ( 'NONE', #8912, #11134, #5313 ) ;
#5388=CIRCLE ( 'NONE', #10806, 5.000000000000004441 ) ;
#5395=EDGE_LOOP ( 'NONE', ( #11149, #11866, #3007, #9629 ) ) ;
#5398=CARTESIAN_POINT ( 'NONE',  ( 642.5000000000001137, 160.0000000000000284, -225.5000000000000000 ) ) ;
#5430=CARTESIAN_POINT ( 'NONE',  ( 639.0000000000000000, 164.0000000000000000, -233.5000000000000000 ) ) ;
#5440=CIRCLE ( 'NONE', #3554, 5.000000000000004441 ) ;
#5444=VECTOR ( 'NONE', #2450, 1000.000000000000114 ) ;
#5453=EDGE_LOOP ( 'NONE', ( #3243, #5815, #2472, #1556 ) ) ;
#5463=CARTESIAN_POINT ( 'NONE',  ( 640.0000000000000000, 160.0000000000000284, -187.5000000000000000 ) ) ;
#5466=DIRECTION ( 'NONE',  ( 0.3543563944859323689, -0.9351104457158684324, 0.000000000000000000 ) ) ;
#5496=DIRECTION ( 'NONE',  ( -1.000000000000000000, 0.000000000000000000, 0.000000000000000000 ) ) ;
#5530=ADVANCED_FACE ( 'NONE', ( #14235, #9796 ), #12973, .F. ) ;
#5541=( NAMED_UNIT ( * ) PLANE_ANGLE_UNIT ( ) SI_UNIT ( $, .RADIAN. ) );
#5546=ORIENTED_EDGE ( 'NONE', *, *, #7454, .T. ) ;
#5553=DIRECTION ( 'NONE',  ( 0.000000000000000000, -0.000000000000000000, 1.000000000000000000 ) ) ;
#5560=ORIENTED_EDGE ( 'NONE', *, *, #10251, .T. ) ;
#5576=CARTESIAN_POINT ( 'NONE',  ( 640.0000000000000000, 160.0000000000000284, 215.5000000000000000 ) ) ;
#5590=CARTESIAN_POINT ( 'NONE',  ( 635.0000000000000000, 160.0000000000000284, -210.0000000000000000 ) ) ;
#5608=ORIENTED_EDGE ( 'NONE', *, *, #5783, .F. ) ;
#5624=EDGE_LOOP ( 'NONE', ( #4777, #1328, #3425, #14458 ) ) ;
#5643=ORIENTED_EDGE ( 'NONE', *, *, #677, .T. ) ;
#5645=DIRECTION ( 'NONE',  ( -1.000000000000000000, 0.000000000000000000, 0.000000000000000000 ) ) ;
#5663=EDGE_LOOP ( 'NONE', ( #6542, #10368, #11385, #5643 ) ) ;
#5687=SHAPE_DEFINITION_REPRESENTATION ( #6309, #9980 ) ;
#5692=VERTEX_POINT ( 'NONE', #8836 ) ;
#5714=DIRECTION ( 'NONE',  ( -1.000000000000000000, 0.000000000000000000, 0.000000000000000000 ) ) ;
#5720=FACE_OUTER_BOUND ( 'NONE', #9989, .T. ) ;
#5734=AXIS2_PLACEMENT_3D ( 'NONE', #7407, #7252, #11893 ) ;
#5741=ORIENTED_EDGE ( 'NONE', *, *, #8812, .F. ) ;
#5763=ADVANCED_FACE ( 'NONE', ( #3439 ), #1363, .F. ) ;
#5765=PRODUCT_DEFINITION ( 'UNKNOWN', '', #515, #8118 ) ;
#5783=EDGE_CURVE ( 'NONE', #4527, #9723, #247, .T. ) ;
#5813=DIRECTION ( 'NONE',  ( 0.000000000000000000, 0.000000000000000000, -1.000000000000000000 ) ) ;
#5815=ORIENTED_EDGE ( 'NONE', *, *, #10063, .F. ) ;
#5825=VECTOR ( 'NONE', #10107, 1000.000000000000000 ) ;
#5828=EDGE_CURVE ( 'NONE', #2732, #7703, #4662, .T. ) ;
#5831=LINE ( 'NONE', #3994, #12906 ) ;
#5843=DIRECTION ( 'NONE',  ( -0.000000000000000000, -0.000000000000000000, -1.000000000000000000 ) ) ;
#5859=AXIS2_PLACEMENT_3D ( 'NONE', #2372, #8057, #2448 ) ;
#5876=CIRCLE ( 'NONE', #14133, 4.799999999999968736 ) ;
#5899=ORIENTED_EDGE ( 'NONE', *, *, #5347, .T. ) ;
#5901=CIRCLE ( 'NONE', #10148, 4.799999999999968736 ) ;
#5966=CARTESIAN_POINT ( 'NONE',  ( 635.0000000000000000, 160.0000000000000284, 210.0000000000000000 ) ) ;
#5974=ORIENTED_EDGE ( 'NONE', *, *, #8181, .T. ) ;
#5993=EDGE_LOOP ( 'NONE', ( #6368, #894, #11400, #8070 ) ) ;
#6001=CARTESIAN_POINT ( 'NONE',  ( 629.0000000000000000, 166.0000000000000284, 187.5000000000000000 ) ) ;
#6004=DIRECTION ( 'NONE',  ( -1.000000000000000000, 0.000000000000000000, 0.000000000000000000 ) ) ;
#6015=DIRECTION ( 'NONE',  ( -0.4113766427172327877, 0.9114654452181378819, 0.000000000000000000 ) ) ;
#6031=ORIENTED_EDGE ( 'NONE', *, *, #3226, .T. ) ;
#6041=ORIENTED_EDGE ( 'NONE', *, *, #1312, .F. ) ;
#6048=EDGE_CURVE ( 'NONE', #7703, #11833, #13837, .T. ) ;
#6053=VERTEX_POINT ( 'NONE', #3716 ) ;
#6092=ORIENTED_EDGE ( 'NONE', *, *, #11301, .F. ) ;
#6098=DIRECTION ( 'NONE',  ( 0.000000000000000000, 0.000000000000000000, -1.000000000000000000 ) ) ;
#6106=EDGE_CURVE ( 'NONE', #5692, #7390, #4677, .T. ) ;
#6107=CARTESIAN_POINT ( 'NONE',  ( 637.5000000000000000, 160.0000000000000284, -233.5000000000000000 ) ) ;
#6114=ORIENTED_EDGE ( 'NONE', *, *, #8516, .F. ) ;
#6117=DIRECTION ( 'NONE',  ( -1.000000000000000000, 0.000000000000000000, 0.000000000000000000 ) ) ;
#6132=VECTOR ( 'NONE', #12094, 1000.000000000000000 ) ;
#6144=ORIENTED_EDGE ( 'NONE', *, *, #11237, .F. ) ;
#6151=LINE ( 'NONE', #11823, #12695 ) ;
#6155=FACE_OUTER_BOUND ( 'NONE', #9889, .T. ) ;
#6198=EDGE_CURVE ( 'NONE', #11788, #2298, #2278, .T. ) ;
#6216=DIRECTION ( 'NONE',  ( 0.000000000000000000, 0.000000000000000000, 1.000000000000000000 ) ) ;
#6220=PLANE ( 'NONE',  #14563 ) ;
#6240=CARTESIAN_POINT ( 'NONE',  ( 636.9746078850427011, 155.6249658629529620, -211.0000000000000000 ) ) ;
#6248=DIRECTION ( 'NONE',  ( 0.3543563944859323134, -0.9351104457158685435, 0.000000000000000000 ) ) ;
#6249=ORIENTED_EDGE ( 'NONE', *, *, #1119, .T. ) ;
#6257=DIRECTION ( 'NONE',  ( -0.000000000000000000, -0.000000000000000000, -1.000000000000000000 ) ) ;
#6268=LINE ( 'NONE', #4074, #12987 ) ;
#6269=LINE ( 'NONE', #11940, #7895 ) ;
#6270=EDGE_LOOP ( 'NONE', ( #255, #9779, #1774, #4210 ) ) ;
#6279=CARTESIAN_POINT ( 'NONE',  ( 636.7009106935324780, 155.5114698605638637, -210.0000000000000000 ) ) ;
#6283=EDGE_CURVE ( 'NONE', #12986, #9079, #3746, .T. ) ;
#6309=PRODUCT_DEFINITION_SHAPE ( 'NONE', 'NONE',  #5765 ) ;
#6321=ORIENTED_EDGE ( 'NONE', *, *, #1048, .F. ) ;
#6348=AXIS2_PLACEMENT_3D ( 'NONE', #13406, #12295, #4709 ) ;
#6359=CARTESIAN_POINT ( 'NONE',  ( 630.0000000000000000, 160.0000000000000284, 215.5000000000000000 ) ) ;
#6368=ORIENTED_EDGE ( 'NONE', *, *, #13088, .T. ) ;
#6408=VERTEX_POINT ( 'NONE', #10898 ) ;
#6413=VERTEX_POINT ( 'NONE', #909 ) ;
#6416=CARTESIAN_POINT ( 'NONE',  ( 635.0000000000000000, 160.0000000000000284, -210.0000000000000000 ) ) ;
#6417=DIRECTION ( 'NONE',  ( 1.000000000000000000, 0.000000000000000000, 0.000000000000000000 ) ) ;
#6433=ORIENTED_EDGE ( 'NONE', *, *, #218, .F. ) ;
#6452=FACE_OUTER_BOUND ( 'NONE', #2186, .T. ) ;
#6462=DIRECTION ( 'NONE',  ( -0.9237280213470676626, -0.3830490080632388272, 0.000000000000000000 ) ) ;
#6474=CARTESIAN_POINT ( 'NONE',  ( 635.0000000000000000, 160.0000000000000284, -222.5000000000000000 ) ) ;
#6479=ORIENTED_EDGE ( 'NONE', *, *, #5828, .F. ) ;
#6506=EDGE_CURVE ( 'NONE', #10347, #2358, #6685, .T. ) ;
#6507=ORIENTED_EDGE ( 'NONE', *, *, #13862, .T. ) ;
#6510=CARTESIAN_POINT ( 'NONE',  ( 636.9746078850427011, 155.6249658629529620, 211.0000000000000000 ) ) ;
#6511=EDGE_CURVE ( 'NONE', #5031, #11833, #13387, .T. ) ;
#6513=ADVANCED_BREP_SHAPE_REPRESENTATION ( '', ( #2557, #9440 ), #9925 ) ;
#6533=CARTESIAN_POINT ( 'NONE',  ( 630.0000000000000000, 160.0000000000000284, 215.5000000000000000 ) ) ;
#6537=CARTESIAN_POINT ( 'NONE',  ( 635.0000000000000000, 160.0000000000000284, -210.0000000000000000 ) ) ;
#6542=ORIENTED_EDGE ( 'NONE', *, *, #1119, .F. ) ;
#6574=ADVANCED_FACE ( 'NONE', ( #12497 ), #2303, .F. ) ;
#6589=PLANE ( 'NONE',  #11047 ) ;
#6594=CIRCLE ( 'NONE', #203, 2.499999999999946709 ) ;
#6633=AXIS2_PLACEMENT_3D ( 'NONE', #14162, #11862, #2871 ) ;
#6638=ADVANCED_FACE ( 'NONE', ( #3366 ), #14570, .F. ) ;
#6647=DIRECTION ( 'NONE',  ( -1.000000000000000000, 0.000000000000000000, 0.000000000000000000 ) ) ;
#6659=ADVANCED_FACE ( 'NONE', ( #11 ), #4548, .F. ) ;
#6667=CARTESIAN_POINT ( 'NONE',  ( 635.0000000000000000, 160.0000000000000284, 187.5000000000000000 ) ) ;
#6685=LINE ( 'NONE', #10001, #4192 ) ;
#6697=ORIENTED_EDGE ( 'NONE', *, *, #7563, .T. ) ;
#6702=ORIENTED_EDGE ( 'NONE', *, *, #8817, .T. ) ;
#6704=ORIENTED_EDGE ( 'NONE', *, *, #6506, .T. ) ;
#6732=LINE ( 'NONE', #4606, #8780 ) ;
#6754=CARTESIAN_POINT ( 'NONE',  ( 641.0000000000000000, 166.0000000000000284, 187.5000000000000000 ) ) ;
#6770=VECTOR ( 'NONE', #6015, 999.9999999999998863 ) ;
#6781=CARTESIAN_POINT ( 'NONE',  ( 636.7009106935324780, 155.5114698605638637, 211.0000000000000000 ) ) ;
#6801=DIRECTION ( 'NONE',  ( 1.000000000000000000, 0.000000000000000000, -0.000000000000000000 ) ) ;
#6806=DIRECTION ( 'NONE',  ( -0.000000000000000000, -0.000000000000000000, -1.000000000000000000 ) ) ;
#6807=ADVANCED_FACE ( 'NONE', ( #6966 ), #1353, .T. ) ;
#6823=DIRECTION ( 'NONE',  ( -0.000000000000000000, -0.000000000000000000, 1.000000000000000000 ) ) ;
#6824=EDGE_LOOP ( 'NONE', ( #11909, #3466, #5608, #5899 ) ) ;
#6830=DIRECTION ( 'NONE',  ( 0.000000000000000000, -1.000000000000000000, 0.000000000000000000 ) ) ;
#6839=ORIENTED_EDGE ( 'NONE', *, *, #11394, .F. ) ;
#6850=DIRECTION ( 'NONE',  ( 1.000000000000000000, 2.312964634635740689E-15, 0.000000000000000000 ) ) ;
#6867=ORIENTED_EDGE ( 'NONE', *, *, #10251, .F. ) ;
#6918=CARTESIAN_POINT ( 'NONE',  ( 630.0000000000000000, 160.0000000000000284, 187.5000000000000000 ) ) ;
#6925=DIRECTION ( 'NONE',  ( -0.000000000000000000, -0.000000000000000000, 1.000000000000000000 ) ) ;
#6938=EDGE_LOOP ( 'NONE', ( #1469, #6704, #602, #10994 ) ) ;
#6943=CARTESIAN_POINT ( 'NONE',  ( 629.0000000000000000, 166.0000000000000284, 187.5000000000000000 ) ) ;
#6951=ADVANCED_FACE ( 'NONE', ( #4734 ), #6589, .F. ) ;
#6965=CARTESIAN_POINT ( 'NONE',  ( 639.4338945024659324, 161.8386352387035743, -210.0000000000000000 ) ) ;
#6966=FACE_OUTER_BOUND ( 'NONE', #531, .T. ) ;
#6975=DIRECTION ( 'NONE',  ( -0.9237280213470676626, -0.3830490080632388272, 0.000000000000000000 ) ) ;
#7022=CARTESIAN_POINT ( 'NONE',  ( 636.7717819724297215, 155.3244477714206653, -222.5000000000000000 ) ) ;
#7027=VECTOR ( 'NONE', #7915, 1000.000000000000000 ) ;
#7042=DIRECTION ( 'NONE',  ( 0.3543563944859323689, -0.9351104457158684324, 0.000000000000000000 ) ) ;
#7047=ORIENTED_EDGE ( 'NONE', *, *, #7972, .T. ) ;
#7063=DIRECTION ( 'NONE',  ( -1.000000000000000000, 0.000000000000000000, 0.000000000000000000 ) ) ;
#7064=CARTESIAN_POINT ( 'NONE',  ( 631.0000000000000000, 164.0000000000000284, -233.5000000000000000 ) ) ;
#7071=ORIENTED_EDGE ( 'NONE', *, *, #11623, .F. ) ;
#7081=ORIENTED_EDGE ( 'NONE', *, *, #6511, .F. ) ;
#7085=AXIS2_PLACEMENT_3D ( 'NONE', #267, #4808, #14021 ) ;
#7091=ORIENTED_EDGE ( 'NONE', *, *, #14497, .F. ) ;
#7102=DIRECTION ( 'NONE',  ( -0.9237280213470676626, -0.3830490080632388272, 0.000000000000000000 ) ) ;
#7127=CIRCLE ( 'NONE', #1938, 2.499999999999946709 ) ;
#7130=DIRECTION ( 'NONE',  ( 0.000000000000000000, 0.000000000000000000, -1.000000000000000000 ) ) ;
#7132=ORIENTED_EDGE ( 'NONE', *, *, #12602, .T. ) ;
#7148=VERTEX_POINT ( 'NONE', #3230 ) ;
#7191=EDGE_CURVE ( 'NONE', #4012, #4648, #4957, .T. ) ;
#7200=CYLINDRICAL_SURFACE ( 'NONE', #2054, 4.799999999999968736 ) ;
#7201=VERTEX_POINT ( 'NONE', #6918 ) ;
#7223=DIRECTION ( 'NONE',  ( -0.000000000000000000, -0.000000000000000000, 1.000000000000000000 ) ) ;
#7234=EDGE_LOOP ( 'NONE', ( #14029, #12856, #10826 ) ) ;
#7242=VERTEX_POINT ( 'NONE', #3387 ) ;
#7252=DIRECTION ( 'NONE',  ( -1.000000000000000000, 0.000000000000000000, 0.000000000000000000 ) ) ;
#7273=CARTESIAN_POINT ( 'NONE',  ( 636.7009106935324780, 155.5114698605638637, 211.0000000000000000 ) ) ;
#7331=CARTESIAN_POINT ( 'NONE',  ( 635.0000000000000000, 160.0000000000000284, -210.0000000000000000 ) ) ;
#7343=CYLINDRICAL_SURFACE ( 'NONE', #4745, 4.799999999999968736 ) ;
#7367=VERTEX_POINT ( 'NONE', #5080 ) ;
#7387=CARTESIAN_POINT ( 'NONE',  ( 641.0000000000000000, 166.0000000000000284, -187.5000000000000000 ) ) ;
#7389=CARTESIAN_POINT ( 'NONE',  ( 635.0000000000000000, 160.0000000000000284, -211.0000000000000000 ) ) ;
#7390=VERTEX_POINT ( 'NONE', #12822 ) ;
#7400=ORIENTED_EDGE ( 'NONE', *, *, #4047, .F. ) ;
#7404=FACE_OUTER_BOUND ( 'NONE', #4742, .T. ) ;
#7407=CARTESIAN_POINT ( 'NONE',  ( 641.0000000000000000, 154.0000000000000568, 187.5000000000000000 ) ) ;
#7414=ORIENTED_EDGE ( 'NONE', *, *, #8258, .T. ) ;
#7419=DIRECTION ( 'NONE',  ( -1.000000000000000000, -6.938893903907222067E-15, 0.000000000000000000 ) ) ;
#7429=DIRECTION ( 'NONE',  ( 1.000000000000000000, 2.312964634635740689E-15, 0.000000000000000000 ) ) ;
#7431=EDGE_LOOP ( 'NONE', ( #2095, #8649, #13672, #3630 ) ) ;
#7452=DIRECTION ( 'NONE',  ( -0.9237280213470676626, -0.3830490080632388272, 0.000000000000000000 ) ) ;
#7454=EDGE_CURVE ( 'NONE', #14292, #30, #5876, .T. ) ;
#7476=LINE ( 'NONE', #2915, #1613 ) ;
#7487=ORIENTED_EDGE ( 'NONE', *, *, #12686, .F. ) ;
#7515=EDGE_LOOP ( 'NONE', ( #7400, #4256, #14109, #6031 ) ) ;
#7516=AXIS2_PLACEMENT_3D ( 'NONE', #2079, #9098, #1114 ) ;
#7527=UNCERTAINTY_MEASURE_WITH_UNIT (LENGTH_MEASURE( 1.000000000000000082E-05 ), #13846, 'distance_accuracy_value', 'NONE');
#7535=DIRECTION ( 'NONE',  ( 0.000000000000000000, 0.000000000000000000, 1.000000000000000000 ) ) ;
#7539=CARTESIAN_POINT ( 'NONE',  ( 635.0000000000000000, 160.0000000000000284, 211.0000000000000000 ) ) ;
#7545=AXIS2_PLACEMENT_3D ( 'NONE', #8816, #3202, #7641 ) ;
#7560=ORIENTED_EDGE ( 'NONE', *, *, #13251, .T. ) ;
#7562=AXIS2_PLACEMENT_3D ( 'NONE', #11732, #13896, #361 ) ;
#7563=EDGE_CURVE ( 'NONE', #4046, #2298, #13477, .T. ) ;
#7568=DIRECTION ( 'NONE',  ( 0.000000000000000000, 0.000000000000000000, -1.000000000000000000 ) ) ;
#7577=ORIENTED_EDGE ( 'NONE', *, *, #7821, .F. ) ;
#7578=AXIS2_PLACEMENT_3D ( 'NONE', #4123, #2867, #11860 ) ;
#7603=DIRECTION ( 'NONE',  ( -0.000000000000000000, -0.000000000000000000, -1.000000000000000000 ) ) ;
#7641=DIRECTION ( 'NONE',  ( -1.000000000000000000, 0.000000000000000000, 0.000000000000000000 ) ) ;
#7680=FACE_OUTER_BOUND ( 'NONE', #10261, .T. ) ;
#7687=VERTEX_POINT ( 'NONE', #375 ) ;
#7692=ORIENTED_EDGE ( 'NONE', *, *, #10333, .T. ) ;
#7698=DIRECTION ( 'NONE',  ( 0.8571673013836776933, 1.049727191973295533E-16, -0.5150380737757388472 ) ) ;
#7701=LINE ( 'NONE', #4105, #10612 ) ;
#7703=VERTEX_POINT ( 'NONE', #11615 ) ;
#7718=EDGE_LOOP ( 'NONE', ( #7047, #509, #8408, #8126 ) ) ;
#7748=FACE_OUTER_BOUND ( 'NONE', #4657, .T. ) ;
#7777=ORIENTED_EDGE ( 'NONE', *, *, #4228, .F. ) ;
#7783=EDGE_LOOP ( 'NONE', ( #2210, #9366 ) ) ;
#7790=DIRECTION ( 'NONE',  ( -1.000000000000000000, 0.000000000000000000, 0.000000000000000000 ) ) ;
#7801=EDGE_LOOP ( 'NONE', ( #11270, #10752 ) ) ;
#7821=EDGE_CURVE ( 'NONE', #5128, #7703, #7701, .T. ) ;
#7823=CIRCLE ( 'NONE', #10182, 7.500000000000062172 ) ;
#7848=LINE ( 'NONE', #12333, #2900 ) ;
#7853=DIRECTION ( 'NONE',  ( -1.000000000000000000, 0.000000000000000000, 0.000000000000000000 ) ) ;
#7869=DIRECTION ( 'NONE',  ( 0.000000000000000000, -0.000000000000000000, -1.000000000000000000 ) ) ;
#7873=ORIENTED_EDGE ( 'NONE', *, *, #11605, .F. ) ;
#7881=LINE ( 'NONE', #12366, #13188 ) ;
#7895=VECTOR ( 'NONE', #9753, 1000.000000000000000 ) ;
#7901=EDGE_CURVE ( 'NONE', #4197, #12301, #2155, .T. ) ;
#7907=ADVANCED_FACE ( 'NONE', ( #13531, #9987 ), #2289, .F. ) ;
#7915=DIRECTION ( 'NONE',  ( -0.000000000000000000, -1.000000000000000000, -0.000000000000000000 ) ) ;
#7925=EDGE_CURVE ( 'NONE', #2358, #7390, #14557, .T. ) ;
#7930=DIRECTION ( 'NONE',  ( 0.000000000000000000, 0.000000000000000000, -1.000000000000000000 ) ) ;
#7931=ORIENTED_EDGE ( 'NONE', *, *, #11301, .T. ) ;
#7948=ORIENTED_EDGE ( 'NONE', *, *, #12602, .F. ) ;
#7950=CARTESIAN_POINT ( 'NONE',  ( 629.0000000000000000, 154.0000000000000284, 187.5000000000000000 ) ) ;
#7958=PLANE ( 'NONE',  #8260 ) ;
#7972=EDGE_CURVE ( 'NONE', #7687, #2732, #6732, .T. ) ;
#7992=LINE ( 'NONE', #13541, #11547 ) ;
#8007=VERTEX_POINT ( 'NONE', #10490 ) ;
#8029=AXIS2_PLACEMENT_3D ( 'NONE', #9435, #4936, #13637 ) ;
#8036=CARTESIAN_POINT ( 'NONE',  ( 0.000000000000000000, 0.000000000000000000, 187.5000000000000000 ) ) ;
#8050=DIRECTION ( 'NONE',  ( 0.000000000000000000, 0.000000000000000000, 1.000000000000000000 ) ) ;
#8057=DIRECTION ( 'NONE',  ( 0.000000000000000000, 0.000000000000000000, 1.000000000000000000 ) ) ;
#8062=ORIENTED_EDGE ( 'NONE', *, *, #1312, .T. ) ;
#8070=ORIENTED_EDGE ( 'NONE', *, *, #11394, .T. ) ;
#8081=EDGE_CURVE ( 'NONE', #9723, #4197, #2512, .T. ) ;
#8083=CARTESIAN_POINT ( 'NONE',  ( 629.0000000000000000, 166.0000000000000284, -187.5000000000000000 ) ) ;
#8093=ORIENTED_EDGE ( 'NONE', *, *, #4583, .F. ) ;
#8118=PRODUCT_DEFINITION_CONTEXT ( 'detailed design', #1508, 'design' ) ;
#8126=ORIENTED_EDGE ( 'NONE', *, *, #1079, .F. ) ;
#8142=VERTEX_POINT ( 'NONE', #10714 ) ;
#8154=CARTESIAN_POINT ( 'NONE',  ( 635.0000000000000000, 160.0000000000000284, -187.5000000000000000 ) ) ;
#8181=EDGE_CURVE ( 'NONE', #8669, #5128, #5901, .T. ) ;
#8182=AXIS2_PLACEMENT_3D ( 'NONE', #3429, #4463, #7869 ) ;
#8188=STYLED_ITEM('',(#14688),#2557);
#8194=ORIENTED_EDGE ( 'NONE', *, *, #1471, .T. ) ;
#8198=DIRECTION ( 'NONE',  ( 1.000000000000000000, 0.000000000000000000, 0.000000000000000000 ) ) ;
#8204=ORIENTED_EDGE ( 'NONE', *, *, #9413, .F. ) ;
#8213=ORIENTED_EDGE ( 'NONE', *, *, #9717, .F. ) ;
#8232=FILL_AREA_STYLE ('',( #9423 ) ) ;
#8239=DIRECTION ( 'NONE',  ( 1.000000000000000000, 0.000000000000000000, 0.000000000000000000 ) ) ;
#8258=EDGE_CURVE ( 'NONE', #14073, #14292, #4496, .T. ) ;
#8260=AXIS2_PLACEMENT_3D ( 'NONE', #8036, #11361, #12450 ) ;
#8281=CIRCLE ( 'NONE', #7545, 2.499999999999946709 ) ;
#8284=DIRECTION ( 'NONE',  ( -0.000000000000000000, -0.000000000000000000, -1.000000000000000000 ) ) ;
#8298=ORIENTED_EDGE ( 'NONE', *, *, #7901, .T. ) ;
#8304=FACE_OUTER_BOUND ( 'NONE', #5395, .T. ) ;
#8311=SURFACE_SIDE_STYLE ('',( #2853 ) ) ;
#8322=DIRECTION ( 'NONE',  ( 0.000000000000000000, 1.000000000000000000, 0.000000000000000000 ) ) ;
#8326=VERTEX_POINT ( 'NONE', #53 ) ;
#8355=CARTESIAN_POINT ( 'NONE',  ( 632.5000000000001137, 160.0000000000000284, -217.5000000000000284 ) ) ;
#8368=LINE ( 'NONE', #9340, #491 ) ;
#8384=CARTESIAN_POINT ( 'NONE',  ( 636.7009106935324780, 155.5114698605638637, -210.0000000000000000 ) ) ;
#8400=CARTESIAN_POINT ( 'NONE',  ( 636.9746078850427011, 155.6249658629529620, 210.0000000000000000 ) ) ;
#8407=LINE ( 'NONE', #13886, #10075 ) ;
#8408=ORIENTED_EDGE ( 'NONE', *, *, #403, .F. ) ;
#8421=AXIS2_PLACEMENT_3D ( 'NONE', #12955, #9499, #7130 ) ;
#8447=CIRCLE ( 'NONE', #4926, 2.499999999999946709 ) ;
#8461=FACE_OUTER_BOUND ( 'NONE', #4833, .T. ) ;
#8465=FACE_OUTER_BOUND ( 'NONE', #14306, .T. ) ;
#8479=CARTESIAN_POINT ( 'NONE',  ( 636.7717819724297215, 155.3244477714206653, 211.0000000000000000 ) ) ;
#8501=CARTESIAN_POINT ( 'NONE',  ( 635.0000000000000000, 160.0000000000000284, -225.5000000000000000 ) ) ;
#8513=DIRECTION ( 'NONE',  ( -0.9237280213470676626, -0.3830490080632388272, 0.000000000000000000 ) ) ;
#8516=EDGE_CURVE ( 'NONE', #12301, #6413, #10544, .T. ) ;
#8518=CIRCLE ( 'NONE', #7562, 5.000000000000004441 ) ;
#8535=CARTESIAN_POINT ( 'NONE',  ( 629.0000000000000000, 154.0000000000000284, -187.5000000000000000 ) ) ;
#8560=CIRCLE ( 'NONE', #10213, 5.000000000000004441 ) ;
#8584=LINE ( 'NONE', #10726, #11595 ) ;
#8590=ORIENTED_EDGE ( 'NONE', *, *, #6048, .F. ) ;
#8616=DIRECTION ( 'NONE',  ( -1.000000000000000000, 0.000000000000000000, 0.000000000000000000 ) ) ;
#8649=ORIENTED_EDGE ( 'NONE', *, *, #4200, .T. ) ;
#8656=DIRECTION ( 'NONE',  ( -0.000000000000000000, -0.000000000000000000, 1.000000000000000000 ) ) ;
#8665=DIRECTION ( 'NONE',  ( -0.000000000000000000, -0.000000000000000000, -1.000000000000000000 ) ) ;
#8669=VERTEX_POINT ( 'NONE', #2025 ) ;
#8675=MECHANICAL_DESIGN_GEOMETRIC_PRESENTATION_REPRESENTATION('',(#8188),#13858);
#8700=DIRECTION ( 'NONE',  ( -0.9237280213470682178, -0.3830490080632377725, 0.000000000000000000 ) ) ;
#8704=CARTESIAN_POINT ( 'NONE',  ( 636.7009106935324780, 155.5114698605638637, 211.0000000000000000 ) ) ;
#8717=ORIENTED_EDGE ( 'NONE', *, *, #13527, .T. ) ;
#8719=LINE ( 'NONE', #6510, #708 ) ;
#8727=VECTOR ( 'NONE', #2223, 1000.000000000000000 ) ;
#8760=ORIENTED_EDGE ( 'NONE', *, *, #3226, .F. ) ;
#8780=VECTOR ( 'NONE', #12260, 1000.000000000000000 ) ;
#8785=CARTESIAN_POINT ( 'NONE',  ( 631.0000000000000000, 155.9999999999999432, -233.5000000000000000 ) ) ;
#8786=EDGE_CURVE ( 'NONE', #13261, #11130, #2400, .T. ) ;
#8787=CARTESIAN_POINT ( 'NONE',  ( 635.0000000000000000, 160.0000000000000284, 215.5000000000000000 ) ) ;
#8788=CARTESIAN_POINT ( 'NONE',  ( 636.9746078850427011, 155.6249658629529620, -210.0000000000000000 ) ) ;
#8794=AXIS2_PLACEMENT_3D ( 'NONE', #11988, #12135, #4253 ) ;
#8812=EDGE_CURVE ( 'NONE', #9079, #5147, #12507, .T. ) ;
#8816=CARTESIAN_POINT ( 'NONE',  ( 635.0000000000000000, 160.0000000000000284, -233.5000000000000000 ) ) ;
#8817=EDGE_CURVE ( 'NONE', #7390, #11788, #4510, .T. ) ;
#8818=FACE_OUTER_BOUND ( 'NONE', #7718, .T. ) ;
#8835=DIRECTION ( 'NONE',  ( -0.000000000000000000, -0.000000000000000000, -1.000000000000000000 ) ) ;
#8836=CARTESIAN_POINT ( 'NONE',  ( 636.7717819724297215, 155.3244477714206653, -210.0000000000000000 ) ) ;
#8879=ORIENTED_EDGE ( 'NONE', *, *, #12581, .T. ) ;
#8888=ORIENTED_EDGE ( 'NONE', *, *, #12305, .F. ) ;
#8893=VECTOR ( 'NONE', #6098, 1000.000000000000000 ) ;
#8898=EDGE_CURVE ( 'NONE', #1513, #10237, #8368, .T. ) ;
#8912=CARTESIAN_POINT ( 'NONE',  ( 635.0000000000000000, 160.0000000000000284, -222.5000000000000000 ) ) ;
#8922=CARTESIAN_POINT ( 'NONE',  ( 635.0000000000000000, 160.0000000000000284, 215.5000000000000000 ) ) ;
#8933=DIRECTION ( 'NONE',  ( -0.9237280213470676626, -0.3830490080632388272, 0.000000000000000000 ) ) ;
#8943=DIRECTION ( 'NONE',  ( -1.000000000000000000, 0.000000000000000000, 0.000000000000000000 ) ) ;
#8944=DIRECTION ( 'NONE',  ( -0.000000000000000000, -0.000000000000000000, -1.000000000000000000 ) ) ;
#8956=AXIS2_PLACEMENT_3D ( 'NONE', #13035, #4917, #7419 ) ;
#8964=DIRECTION ( 'NONE',  ( -0.000000000000000000, -0.000000000000000000, -1.000000000000000000 ) ) ;
#8974=VECTOR ( 'NONE', #7568, 1000.000000000000000 ) ;
#8986=DIRECTION ( 'NONE',  ( -1.000000000000000000, 0.000000000000000000, 0.000000000000000000 ) ) ;
#9010=EDGE_CURVE ( 'NONE', #9101, #12192, #10172, .T. ) ;
#9034=ORIENTED_EDGE ( 'NONE', *, *, #2021, .T. ) ;
#9065=EDGE_CURVE ( 'NONE', #11130, #9710, #8281, .T. ) ;
#9071=DIRECTION ( 'NONE',  ( 1.000000000000000000, -3.469446951953611033E-15, 0.000000000000000000 ) ) ;
#9079=VERTEX_POINT ( 'NONE', #682 ) ;
#9098=DIRECTION ( 'NONE',  ( -0.9114654452181378819, -0.4113766427172328988, 0.000000000000000000 ) ) ;
#9101=VERTEX_POINT ( 'NONE', #2010 ) ;
#9111=VERTEX_POINT ( 'NONE', #3060 ) ;
#9116=CARTESIAN_POINT ( 'NONE',  ( 630.0000000000000000, 160.0000000000000284, -187.5000000000000000 ) ) ;
#9129=DIRECTION ( 'NONE',  ( 0.000000000000000000, 0.000000000000000000, -1.000000000000000000 ) ) ;
#9176=ORIENTED_EDGE ( 'NONE', *, *, #7901, .F. ) ;
#9177=ORIENTED_EDGE ( 'NONE', *, *, #11085, .T. ) ;
#9190=ADVANCED_FACE ( 'NONE', ( #3649 ), #1278, .T. ) ;
#9212=FACE_BOUND ( 'NONE', #10790, .T. ) ;
#9257=EDGE_LOOP ( 'NONE', ( #11233, #6433 ) ) ;
#9302=CARTESIAN_POINT ( 'NONE',  ( 639.0000000000000000, 156.0000000000000000, -225.5000000000000000 ) ) ;
#9315=CARTESIAN_POINT ( 'NONE',  ( 635.0000000000000000, 160.0000000000000284, 210.0000000000000000 ) ) ;
#9320=ORIENTED_EDGE ( 'NONE', *, *, #14048, .F. ) ;
#9340=CARTESIAN_POINT ( 'NONE',  ( 641.0000000000000000, 154.0000000000000568, -187.5000000000000000 ) ) ;
#9343=DIRECTION ( 'NONE',  ( -0.9237280213470676626, -0.3830490080632388272, 0.000000000000000000 ) ) ;
#9354=DIRECTION ( 'NONE',  ( -1.000000000000000000, 0.000000000000000000, -0.000000000000000000 ) ) ;
#9356=ADVANCED_FACE ( 'NONE', ( #4830 ), #3717, .T. ) ;
#9366=ORIENTED_EDGE ( 'NONE', *, *, #11237, .T. ) ;
#9385=AXIS2_PLACEMENT_3D ( 'NONE', #7331, #10661, #9486 ) ;
#9413=EDGE_CURVE ( 'NONE', #11816, #12048, #8518, .T. ) ;
#9414=CARTESIAN_POINT ( 'NONE',  ( 629.0000000000000000, 154.0000000000000284, 187.5000000000000000 ) ) ;
#9423=FILL_AREA_STYLE_COLOUR ( '', #9699 ) ;
#9435=CARTESIAN_POINT ( 'NONE',  ( 635.0000000000000000, 160.0000000000000284, -222.5000000000000000 ) ) ;
#9440=AXIS2_PLACEMENT_3D ( 'NONE', #4347, #14302, #6417 ) ;
#9447=LINE ( 'NONE', #2720, #11253 ) ;
#9448=ORIENTED_EDGE ( 'NONE', *, *, #14247, .T. ) ;
#9462=DIRECTION ( 'NONE',  ( 0.000000000000000000, 0.000000000000000000, 1.000000000000000000 ) ) ;
#9465=EDGE_CURVE ( 'NONE', #8669, #2732, #8719, .T. ) ;
#9486=DIRECTION ( 'NONE',  ( -1.000000000000000000, 0.000000000000000000, 0.000000000000000000 ) ) ;
#9499=DIRECTION ( 'NONE',  ( 1.000000000000000000, -0.000000000000000000, 0.000000000000000000 ) ) ;
#9506=CIRCLE ( 'NONE', #3142, 5.000000000000004441 ) ;
#9512=EDGE_CURVE ( 'NONE', #12112, #6053, #3120, .T. ) ;
#9540=ADVANCED_FACE ( 'NONE', ( #9827 ), #10783, .T. ) ;
#9543=VERTEX_POINT ( 'NONE', #11074 ) ;
#9565=FACE_OUTER_BOUND ( 'NONE', #5074, .T. ) ;
#9606=ORIENTED_EDGE ( 'NONE', *, *, #12686, .T. ) ;
#9629=ORIENTED_EDGE ( 'NONE', *, *, #2151, .T. ) ;
#9647=EDGE_CURVE ( 'NONE', #12192, #2358, #4255, .T. ) ;
#9662=CARTESIAN_POINT ( 'NONE',  ( 635.0000000000000000, 160.0000000000000284, -217.5000000000000284 ) ) ;
#9676=VECTOR ( 'NONE', #11889, 1000.000000000000000 ) ;
#9699=COLOUR_RGB ( '',0.8941176470588234615, 0.8941176470588234615, 0.8941176470588234615 ) ;
#9700=DIRECTION ( 'NONE',  ( -0.9237280213470682178, -0.3830490080632377725, 0.000000000000000000 ) ) ;
#9702=CARTESIAN_POINT ( 'NONE',  ( 635.0000000000000000, 160.0000000000000284, 211.0000000000000000 ) ) ;
#9710=VERTEX_POINT ( 'NONE', #11152 ) ;
#9717=EDGE_CURVE ( 'NONE', #9543, #344, #1656, .T. ) ;
#9719=DIRECTION ( 'NONE',  ( 0.000000000000000000, 0.000000000000000000, 1.000000000000000000 ) ) ;
#9723=VERTEX_POINT ( 'NONE', #3472 ) ;
#9745=ORIENTED_EDGE ( 'NONE', *, *, #12861, .T. ) ;
#9753=DIRECTION ( 'NONE',  ( -0.000000000000000000, -0.000000000000000000, -1.000000000000000000 ) ) ;
#9768=FACE_OUTER_BOUND ( 'NONE', #13738, .T. ) ;
#9770=DIRECTION ( 'NONE',  ( -0.000000000000000000, -0.000000000000000000, -1.000000000000000000 ) ) ;
#9774=DIRECTION ( 'NONE',  ( 0.000000000000000000, 0.000000000000000000, -1.000000000000000000 ) ) ;
#9779=ORIENTED_EDGE ( 'NONE', *, *, #4907, .T. ) ;
#9780=CARTESIAN_POINT ( 'NONE',  ( 635.0000000000000000, 160.0000000000000284, -211.0000000000000000 ) ) ;
#9796=FACE_OUTER_BOUND ( 'NONE', #10944, .T. ) ;
#9805=CARTESIAN_POINT ( 'NONE',  ( 630.0000000000000000, 160.0000000000000284, -210.0000000000000000 ) ) ;
#9827=FACE_OUTER_BOUND ( 'NONE', #11434, .T. ) ;
#9836=AXIS2_PLACEMENT_3D ( 'NONE', #1343, #3648, #7102 ) ;
#9849=VERTEX_POINT ( 'NONE', #4438 ) ;
#9853=FACE_OUTER_BOUND ( 'NONE', #11092, .T. ) ;
#9889=EDGE_LOOP ( 'NONE', ( #4342, #917, #7777, #23 ) ) ;
#9902=AXIS2_PLACEMENT_3D ( 'NONE', #4660, #12391, #2360 ) ;
#9920=VECTOR ( 'NONE', #5466, 1000.000000000000227 ) ;
#9925=( GEOMETRIC_REPRESENTATION_CONTEXT ( 3 ) GLOBAL_UNCERTAINTY_ASSIGNED_CONTEXT ( ( #7527 ) ) GLOBAL_UNIT_ASSIGNED_CONTEXT ( ( #13846, #11848, #5078 ) ) REPRESENTATION_CONTEXT ( 'NONE', 'WORKASPACE' ) );
#9957=ORIENTED_EDGE ( 'NONE', *, *, #7563, .F. ) ;
#9971=PRODUCT_CONTEXT ( 'NONE', #14615, 'mechanical' ) ;
#9980=SHAPE_REPRESENTATION ( 'hub', ( #9440 ), #9925 ) ;
#9981=DIRECTION ( 'NONE',  ( -0.000000000000000000, 0.000000000000000000, -1.000000000000000000 ) ) ;
#9987=FACE_OUTER_BOUND ( 'NONE', #13866, .T. ) ;
#9989=EDGE_LOOP ( 'NONE', ( #8213, #2579, #207, #6321 ) ) ;
#10000=CARTESIAN_POINT ( 'NONE',  ( 637.0568832135862749, 155.4426727739092655, 215.5000000000000000 ) ) ;
#10001=CARTESIAN_POINT ( 'NONE',  ( 636.7009106935324780, 155.5114698605638637, -210.0000000000000000 ) ) ;
#10003=ORIENTED_EDGE ( 'NONE', *, *, #8081, .F. ) ;
#10031=LINE ( 'NONE', #14536, #5825 ) ;
#10057=ORIENTED_EDGE ( 'NONE', *, *, #12495, .F. ) ;
#10063=EDGE_CURVE ( 'NONE', #14073, #8007, #2281, .T. ) ;
#10072=DIRECTION ( 'NONE',  ( -0.000000000000000000, -0.000000000000000000, -1.000000000000000000 ) ) ;
#10075=VECTOR ( 'NONE', #3783, 1000.000000000000000 ) ;
#10105=VECTOR ( 'NONE', #10609, 1000.000000000000000 ) ;
#10106=VECTOR ( 'NONE', #7429, 1000.000000000000000 ) ;
#10107=DIRECTION ( 'NONE',  ( 0.000000000000000000, 1.000000000000000000, 0.000000000000000000 ) ) ;
#10148=AXIS2_PLACEMENT_3D ( 'NONE', #4295, #7535, #1773 ) ;
#10172=CIRCLE ( 'NONE', #11312, 4.799999999999968736 ) ;
#10182=AXIS2_PLACEMENT_3D ( 'NONE', #4615, #146, #5714 ) ;
#10213=AXIS2_PLACEMENT_3D ( 'NONE', #10222, #12804, #2532 ) ;
#10214=CARTESIAN_POINT ( 'NONE',  ( 630.5661054975340676, 158.1613647612965110, 211.0000000000000000 ) ) ;
#10222=CARTESIAN_POINT ( 'NONE',  ( 635.0000000000000000, 160.0000000000000284, 210.0000000000000000 ) ) ;
#10237=VERTEX_POINT ( 'NONE', #7387 ) ;
#10247=EDGE_CURVE ( 'NONE', #9111, #4012, #514, .T. ) ;
#10251=EDGE_CURVE ( 'NONE', #6408, #11788, #6268, .T. ) ;
#10261=EDGE_LOOP ( 'NONE', ( #13519, #6249, #4635, #5027 ) ) ;
#10294=DIRECTION ( 'NONE',  ( 0.000000000000000000, 0.000000000000000000, -1.000000000000000000 ) ) ;
#10307=AXIS2_PLACEMENT_3D ( 'NONE', #11265, #1075, #8986 ) ;
#10318=FACE_OUTER_BOUND ( 'NONE', #6824, .T. ) ;
#10328=CIRCLE ( 'NONE', #9385, 5.000000000000004441 ) ;
#10333=EDGE_CURVE ( 'NONE', #12986, #2721, #14314, .T. ) ;
#10347=VERTEX_POINT ( 'NONE', #1919 ) ;
#10351=AXIS2_PLACEMENT_3D ( 'NONE', #11943, #13142, #2896 ) ;
#10368=ORIENTED_EDGE ( 'NONE', *, *, #8258, .F. ) ;
#10370=AXIS2_PLACEMENT_3D ( 'NONE', #10750, #5234, #5149 ) ;
#10372=LINE ( 'NONE', #8083, #13681 ) ;
#10373=DIRECTION ( 'NONE',  ( -1.000000000000000000, -2.312964634635740689E-15, 0.000000000000000000 ) ) ;
#10385=EDGE_CURVE ( 'NONE', #344, #9543, #11792, .T. ) ;
#10388=ORIENTED_EDGE ( 'NONE', *, *, #3755, .F. ) ;
#10396=VECTOR ( 'NONE', #6925, 1000.000000000000000 ) ;
#10399=EDGE_CURVE ( 'NONE', #13395, #3660, #865, .T. ) ;
#10401=FACE_BOUND ( 'NONE', #9257, .T. ) ;
#10428=DIRECTION ( 'NONE',  ( 0.000000000000000000, 0.000000000000000000, -1.000000000000000000 ) ) ;
#10437=DIRECTION ( 'NONE',  ( -1.000000000000000000, 0.000000000000000000, 0.000000000000000000 ) ) ;
#10466=PLANE ( 'NONE',  #14347 ) ;
#10479=DIRECTION ( 'NONE',  ( -1.000000000000000000, -6.938893903907222067E-15, 0.000000000000000000 ) ) ;
#10490=CARTESIAN_POINT ( 'NONE',  ( 636.9746078850427011, 155.6249658629529620, -211.0000000000000000 ) ) ;
#10500=CARTESIAN_POINT ( 'NONE',  ( 635.0000000000000000, 160.0000000000000284, 210.0000000000000000 ) ) ;
#10506=EDGE_LOOP ( 'NONE', ( #4411, #11879, #1042, #2909 ) ) ;
#10508=ORIENTED_EDGE ( 'NONE', *, *, #7972, .F. ) ;
#10519=CARTESIAN_POINT ( 'NONE',  ( 629.0000000000000000, 154.0000000000000284, 187.5000000000000000 ) ) ;
#10522=SURFACE_STYLE_USAGE ( .BOTH. , #8311 ) ;
#10544=LINE ( 'NONE', #9302, #4992 ) ;
#10577=ADVANCED_FACE ( 'NONE', ( #8465 ), #2650, .F. ) ;
#10594=ORIENTED_EDGE ( 'NONE', *, *, #6283, .F. ) ;
#10600=( NAMED_UNIT ( * ) PLANE_ANGLE_UNIT ( ) SI_UNIT ( $, .RADIAN. ) );
#10607=CIRCLE ( 'NONE', #1164, 4.799999999999968736 ) ;
#10609=DIRECTION ( 'NONE',  ( -0.000000000000000000, -0.000000000000000000, -1.000000000000000000 ) ) ;
#10612=VECTOR ( 'NONE', #14212, 1000.000000000000000 ) ;
#10637=UNCERTAINTY_MEASURE_WITH_UNIT (LENGTH_MEASURE( 1.000000000000000082E-05 ), #390, 'distance_accuracy_value', 'NONE');
#10661=DIRECTION ( 'NONE',  ( 0.000000000000000000, 0.000000000000000000, -1.000000000000000000 ) ) ;
#10683=LINE ( 'NONE', #8535, #10106 ) ;
#10714=CARTESIAN_POINT ( 'NONE',  ( 627.5000000000000000, 160.0000000000000284, -222.5000000000000000 ) ) ;
#10726=CARTESIAN_POINT ( 'NONE',  ( 629.0000000000000000, 154.0000000000000284, 187.5000000000000000 ) ) ;
#10732=ORIENTED_EDGE ( 'NONE', *, *, #403, .T. ) ;
#10748=ORIENTED_EDGE ( 'NONE', *, *, #218, .T. ) ;
#10750=CARTESIAN_POINT ( 'NONE',  ( 636.7009106935324780, 155.5114698605638637, 211.0000000000000000 ) ) ;
#10752=ORIENTED_EDGE ( 'NONE', *, *, #2786, .T. ) ;
#10769=DIRECTION ( 'NONE',  ( -0.000000000000000000, -0.000000000000000000, 1.000000000000000000 ) ) ;
#10783=CYLINDRICAL_SURFACE ( 'NONE', #14384, 4.799999999999968736 ) ;
#10788=CARTESIAN_POINT ( 'NONE',  ( 635.0000000000000000, 160.0000000000000284, 215.5000000000000000 ) ) ;
#10790=EDGE_LOOP ( 'NONE', ( #3812, #2313 ) ) ;
#10806=AXIS2_PLACEMENT_3D ( 'NONE', #5276, #1944, #12117 ) ;
#10826=ORIENTED_EDGE ( 'NONE', *, *, #11605, .T. ) ;
#10855=AXIS2_PLACEMENT_3D ( 'NONE', #13438, #8050, #8933 ) ;
#10864=AXIS2_PLACEMENT_3D ( 'NONE', #9702, #2124, #6647 ) ;
#10872=VECTOR ( 'NONE', #10072, 1000.000000000000000 ) ;
#10876=CARTESIAN_POINT ( 'NONE',  ( 635.0000000000000000, 160.0000000000000284, -211.0000000000000000 ) ) ;
#10880=CARTESIAN_POINT ( 'NONE',  ( 635.0000000000000000, 160.0000000000000284, -225.5000000000000000 ) ) ;
#10890=LINE ( 'NONE', #4169, #2628 ) ;
#10898=CARTESIAN_POINT ( 'NONE',  ( 630.0000000000000000, 160.0000000000000284, -222.5000000000000000 ) ) ;
#10922=ORIENTED_EDGE ( 'NONE', *, *, #14497, .T. ) ;
#10924=PLANE ( 'NONE',  #11975 ) ;
#10942=UNCERTAINTY_MEASURE_WITH_UNIT (LENGTH_MEASURE( 1.000000000000000082E-05 ), #4299, 'distance_accuracy_value', 'NONE');
#10944=EDGE_LOOP ( 'NONE', ( #8760, #11634 ) ) ;
#10945=CARTESIAN_POINT ( 'NONE',  ( 641.0000000000000000, 154.0000000000000568, -187.5000000000000000 ) ) ;
#10980=ORIENTED_EDGE ( 'NONE', *, *, #1602, .T. ) ;
#10981=ORIENTED_EDGE ( 'NONE', *, *, #8516, .T. ) ;
#10994=ORIENTED_EDGE ( 'NONE', *, *, #6106, .F. ) ;
#11002=PLANE ( 'NONE',  #12309 ) ;
#11015=ORIENTED_EDGE ( 'NONE', *, *, #14296, .F. ) ;
#11039=AXIS2_PLACEMENT_3D ( 'NONE', #5966, #101, #3615 ) ;
#11047=AXIS2_PLACEMENT_3D ( 'NONE', #14487, #4584, #11365 ) ;
#11062=CARTESIAN_POINT ( 'NONE',  ( 635.0000000000000000, 160.0000000000000284, -210.0000000000000000 ) ) ;
#11074=CARTESIAN_POINT ( 'NONE',  ( 640.0000000000000000, 160.0000000000000284, 215.5000000000000000 ) ) ;
#11085=EDGE_CURVE ( 'NONE', #7201, #4236, #5015, .T. ) ;
#11092=EDGE_LOOP ( 'NONE', ( #13958, #33, #12584, #10732, #5974, #11403, #7132, #7692 ) ) ;
#11099=MECHANICAL_DESIGN_GEOMETRIC_PRESENTATION_REPRESENTATION('',(#3565),#11113);
#11107=LINE ( 'NONE', #10000, #3259 ) ;
#11113=( GEOMETRIC_REPRESENTATION_CONTEXT ( 3 ) GLOBAL_UNCERTAINTY_ASSIGNED_CONTEXT ( ( #10637 ) ) GLOBAL_UNIT_ASSIGNED_CONTEXT ( ( #390, #10600, #482 ) ) REPRESENTATION_CONTEXT ( 'NONE', 'WORKASPACE' ) );
#11115=ORIENTED_EDGE ( 'NONE', *, *, #3833, .T. ) ;
#11130=VERTEX_POINT ( 'NONE', #904 ) ;
#11134=DIRECTION ( 'NONE',  ( 0.000000000000000000, 0.000000000000000000, -1.000000000000000000 ) ) ;
#11148=CLOSED_SHELL ( 'NONE', ( #3235, #11692, #12396, #14529, #9540, #745, #4795, #13226, #5363, #12224, #9190, #13273, #13324, #10577, #5763, #38, #6638, #14415, #2937, #14283, #5301, #2481, #2884, #206, #2316, #3177, #4349, #12108, #6951, #6807, #9356, #2945, #5530, #2336, #14513, #6659, #4718, #7907, #6574, #12680 ) ) ;
#11149=ORIENTED_EDGE ( 'NONE', *, *, #11623, .T. ) ;
#11152=CARTESIAN_POINT ( 'NONE',  ( 637.5000000000000000, 160.0000000000000284, -233.5000000000000000 ) ) ;
#11160=DIRECTION ( 'NONE',  ( 1.000000000000000000, 0.000000000000000000, 0.000000000000000000 ) ) ;
#11178=CARTESIAN_POINT ( 'NONE',  ( 636.9746078850427011, 155.6249658629529620, -210.0000000000000000 ) ) ;
#11181=DIRECTION ( 'NONE',  ( -0.000000000000000000, -0.000000000000000000, -1.000000000000000000 ) ) ;
#11201=DIRECTION ( 'NONE',  ( -0.000000000000000000, 0.000000000000000000, -1.000000000000000000 ) ) ;
#11204=AXIS2_PLACEMENT_3D ( 'NONE', #5102, #9462, #14100 ) ;
#11233=ORIENTED_EDGE ( 'NONE', *, *, #11085, .F. ) ;
#11237=EDGE_CURVE ( 'NONE', #1071, #12112, #7823, .T. ) ;
#11253=VECTOR ( 'NONE', #7223, 1000.000000000000000 ) ;
#11265=CARTESIAN_POINT ( 'NONE',  ( 635.0000000000000000, 160.0000000000000284, -211.0000000000000000 ) ) ;
#11270=ORIENTED_EDGE ( 'NONE', *, *, #4137, .T. ) ;
#11278=EDGE_CURVE ( 'NONE', #3772, #13817, #11609, .T. ) ;
#11281=DIRECTION ( 'NONE',  ( -0.9237280213470676626, -0.3830490080632388272, 0.000000000000000000 ) ) ;
#11301=EDGE_CURVE ( 'NONE', #5147, #9849, #13717, .T. ) ;
#11311=CARTESIAN_POINT ( 'NONE',  ( 635.0000000000000000, 160.0000000000000284, -217.5000000000000284 ) ) ;
#11312=AXIS2_PLACEMENT_3D ( 'NONE', #9780, #3268, #6462 ) ;
#11320=DIRECTION ( 'NONE',  ( 0.000000000000000000, 0.000000000000000000, 1.000000000000000000 ) ) ;
#11361=DIRECTION ( 'NONE',  ( -0.000000000000000000, 0.000000000000000000, 1.000000000000000000 ) ) ;
#11365=DIRECTION ( 'NONE',  ( -0.9237280213470682178, -0.3830490080632377725, 0.000000000000000000 ) ) ;
#11375=LINE ( 'NONE', #2583, #4717 ) ;
#11385=ORIENTED_EDGE ( 'NONE', *, *, #10063, .T. ) ;
#11394=EDGE_CURVE ( 'NONE', #13817, #11698, #8584, .T. ) ;
#11395=DIRECTION ( 'NONE',  ( -0.9237280213470676626, -0.3830490080632388272, 0.000000000000000000 ) ) ;
#11400=ORIENTED_EDGE ( 'NONE', *, *, #4200, .F. ) ;
#11403=ORIENTED_EDGE ( 'NONE', *, *, #13968, .T. ) ;
#11408=ORIENTED_EDGE ( 'NONE', *, *, #1295, .F. ) ;
#11418=ORIENTED_EDGE ( 'NONE', *, *, #9065, .F. ) ;
#11421=CYLINDRICAL_SURFACE ( 'NONE', #8029, 5.000000000000004441 ) ;
#11434=EDGE_LOOP ( 'NONE', ( #7948, #2625, #1999, #10594 ) ) ;
#11461=CARTESIAN_POINT ( 'NONE',  ( 630.5661054975340676, 158.1613647612965110, -211.0000000000000000 ) ) ;
#11476=ORIENTED_EDGE ( 'NONE', *, *, #3153, .T. ) ;
#11492=FACE_OUTER_BOUND ( 'NONE', #1450, .T. ) ;
#11507=CARTESIAN_POINT ( 'NONE',  ( 637.0568832135862749, 155.4426727739092655, -222.5000000000000000 ) ) ;
#11547=VECTOR ( 'NONE', #12494, 1000.000000000000000 ) ;
#11566=DIRECTION ( 'NONE',  ( -0.9114654452181378819, -0.4113766427172327877, 0.000000000000000000 ) ) ;
#11595=VECTOR ( 'NONE', #13019, 1000.000000000000000 ) ;
#11601=CARTESIAN_POINT ( 'NONE',  ( 635.0000000000000000, 160.0000000000000284, -225.5000000000000000 ) ) ;
#11605=EDGE_CURVE ( 'NONE', #3214, #13261, #7127, .T. ) ;
#11609=LINE ( 'NONE', #6001, #512 ) ;
#11615=CARTESIAN_POINT ( 'NONE',  ( 639.4338945024659324, 161.8386352387035743, 210.0000000000000000 ) ) ;
#11618=AXIS2_PLACEMENT_3D ( 'NONE', #231, #11181, #2464 ) ;
#11619=DIRECTION ( 'NONE',  ( 0.000000000000000000, 1.000000000000000000, 0.000000000000000000 ) ) ;
#11623=EDGE_CURVE ( 'NONE', #6413, #13395, #4060, .T. ) ;
#11634=ORIENTED_EDGE ( 'NONE', *, *, #1471, .F. ) ;
#11640=CARTESIAN_POINT ( 'NONE',  ( 635.0000000000000000, 160.0000000000000284, -233.5000000000000000 ) ) ;
#11657=CARTESIAN_POINT ( 'NONE',  ( 641.0000000000000000, 154.0000000000000568, 187.5000000000000000 ) ) ;
#11687=DIRECTION ( 'NONE',  ( 0.000000000000000000, 0.000000000000000000, -1.000000000000000000 ) ) ;
#11692=ADVANCED_FACE ( 'NONE', ( #11706 ), #1604, .F. ) ;
#11698=VERTEX_POINT ( 'NONE', #14020 ) ;
#11706=FACE_OUTER_BOUND ( 'NONE', #4535, .T. ) ;
#11729=ORIENTED_EDGE ( 'NONE', *, *, #7925, .F. ) ;
#11732=CARTESIAN_POINT ( 'NONE',  ( 635.0000000000000000, 160.0000000000000284, 211.0000000000000000 ) ) ;
#11788=VERTEX_POINT ( 'NONE', #4410 ) ;
#11792=CIRCLE ( 'NONE', #1196, 5.000000000000004441 ) ;
#11799=EDGE_CURVE ( 'NONE', #5692, #2242, #1720, .T. ) ;
#11816=VERTEX_POINT ( 'NONE', #792 ) ;
#11823=CARTESIAN_POINT ( 'NONE',  ( 632.5000000000001137, 160.0000000000000284, -217.5000000000000284 ) ) ;
#11833=VERTEX_POINT ( 'NONE', #12085 ) ;
#11848=( NAMED_UNIT ( * ) PLANE_ANGLE_UNIT ( ) SI_UNIT ( $, .RADIAN. ) );
#11860=DIRECTION ( 'NONE',  ( -1.000000000000000000, 0.000000000000000000, -0.000000000000000000 ) ) ;
#11862=DIRECTION ( 'NONE',  ( 1.000000000000000000, 0.000000000000000000, -0.000000000000000000 ) ) ;
#11866=ORIENTED_EDGE ( 'NONE', *, *, #5347, .F. ) ;
#11879=ORIENTED_EDGE ( 'NONE', *, *, #302, .T. ) ;
#11887=EDGE_LOOP ( 'NONE', ( #9606, #9176, #10003, #6507 ) ) ;
#11889=DIRECTION ( 'NONE',  ( -0.000000000000000000, -0.000000000000000000, 1.000000000000000000 ) ) ;
#11893=DIRECTION ( 'NONE',  ( 0.000000000000000000, 0.000000000000000000, 1.000000000000000000 ) ) ;
#11909=ORIENTED_EDGE ( 'NONE', *, *, #10399, .T. ) ;
#11918=CARTESIAN_POINT ( 'NONE',  ( 641.0000000000000000, 154.0000000000000568, 187.5000000000000000 ) ) ;
#11940=CARTESIAN_POINT ( 'NONE',  ( 641.0000000000000000, 154.0000000000000568, 187.5000000000000000 ) ) ;
#11943=CARTESIAN_POINT ( 'NONE',  ( 635.0000000000000000, 160.0000000000000284, -210.0000000000000000 ) ) ;
#11948=ORIENTED_EDGE ( 'NONE', *, *, #677, .F. ) ;
#11950=DIRECTION ( 'NONE',  ( 0.3543563944859322579, -0.9351104457158685435, 0.000000000000000000 ) ) ;
#11975=AXIS2_PLACEMENT_3D ( 'NONE', #5590, #11201, #8700 ) ;
#11988=CARTESIAN_POINT ( 'NONE',  ( 635.0000000000000000, 160.0000000000000284, 211.0000000000000000 ) ) ;
#12036=AXIS2_PLACEMENT_3D ( 'NONE', #14579, #10294, #5645 ) ;
#12040=ORIENTED_EDGE ( 'NONE', *, *, #10385, .T. ) ;
#12048=VERTEX_POINT ( 'NONE', #12962 ) ;
#12061=ORIENTED_EDGE ( 'NONE', *, *, #9065, .T. ) ;
#12071=FACE_OUTER_BOUND ( 'NONE', #13266, .T. ) ;
#12074=AXIS2_PLACEMENT_3D ( 'NONE', #11640, #2787, #6117 ) ;
#12079=LINE ( 'NONE', #5576, #12476 ) ;
#12085=CARTESIAN_POINT ( 'NONE',  ( 630.5661054975340676, 158.1613647612965110, 210.0000000000000000 ) ) ;
#12094=DIRECTION ( 'NONE',  ( -0.000000000000000000, -0.000000000000000000, 1.000000000000000000 ) ) ;
#12099=ORIENTED_EDGE ( 'NONE', *, *, #6106, .T. ) ;
#12108=ADVANCED_FACE ( 'NONE', ( #9853 ), #991, .T. ) ;
#12112=VERTEX_POINT ( 'NONE', #13108 ) ;
#12114=VERTEX_POINT ( 'NONE', #4175 ) ;
#12117=DIRECTION ( 'NONE',  ( -1.000000000000000000, 0.000000000000000000, 0.000000000000000000 ) ) ;
#12135=DIRECTION ( 'NONE',  ( -0.000000000000000000, 0.000000000000000000, -1.000000000000000000 ) ) ;
#12144=CARTESIAN_POINT ( 'NONE',  ( 631.0000000000000000, 164.0000000000000284, -233.5000000000000000 ) ) ;
#12162=CYLINDRICAL_SURFACE ( 'NONE', #2272, 4.799999999999968736 ) ;
#12180=DIRECTION ( 'NONE',  ( 0.000000000000000000, 0.000000000000000000, -1.000000000000000000 ) ) ;
#12191=ORIENTED_EDGE ( 'NONE', *, *, #10333, .F. ) ;
#12192=VERTEX_POINT ( 'NONE', #11461 ) ;
#12201=CIRCLE ( 'NONE', #13394, 7.500000000000062172 ) ;
#12208=CIRCLE ( 'NONE', #5859, 4.799999999999968736 ) ;
#12224=ADVANCED_FACE ( 'NONE', ( #5720 ), #13544, .T. ) ;
#12233=DIRECTION ( 'NONE',  ( 1.000000000000000000, 0.000000000000000000, -0.000000000000000000 ) ) ;
#12235=ORIENTED_EDGE ( 'NONE', *, *, #1048, .T. ) ;
#12255=DIRECTION ( 'NONE',  ( 0.000000000000000000, 0.000000000000000000, 1.000000000000000000 ) ) ;
#12260=DIRECTION ( 'NONE',  ( -0.4113766427172328433, 0.9114654452181377708, 0.000000000000000000 ) ) ;
#12271=VECTOR ( 'NONE', #4358, 1000.000000000000000 ) ;
#12295=DIRECTION ( 'NONE',  ( 0.000000000000000000, 0.000000000000000000, -1.000000000000000000 ) ) ;
#12301=VERTEX_POINT ( 'NONE', #12942 ) ;
#12305=EDGE_CURVE ( 'NONE', #7148, #7687, #8560, .T. ) ;
#12309=AXIS2_PLACEMENT_3D ( 'NONE', #10876, #9981, #9700 ) ;
#12333=CARTESIAN_POINT ( 'NONE',  ( 630.0000000000000000, 160.0000000000000284, -222.5000000000000000 ) ) ;
#12336=DIRECTION ( 'NONE',  ( 0.000000000000000000, 0.000000000000000000, -1.000000000000000000 ) ) ;
#12366=CARTESIAN_POINT ( 'NONE',  ( 636.9746078850427011, 155.6249658629529620, -210.0000000000000000 ) ) ;
#12377=LINE ( 'NONE', #14464, #6132 ) ;
#12391=DIRECTION ( 'NONE',  ( 0.000000000000000000, 0.000000000000000000, 1.000000000000000000 ) ) ;
#12396=ADVANCED_FACE ( 'NONE', ( #4910 ), #5123, .T. ) ;
#12404=ORIENTED_EDGE ( 'NONE', *, *, #11278, .F. ) ;
#12407=CARTESIAN_POINT ( 'NONE',  ( 635.0000000000000000, 160.0000000000000284, -222.5000000000000000 ) ) ;
#12417=CARTESIAN_POINT ( 'NONE',  ( 635.0000000000000000, 160.0000000000000284, 211.0000000000000000 ) ) ;
#12450=DIRECTION ( 'NONE',  ( 1.000000000000000000, 0.000000000000000000, 0.000000000000000000 ) ) ;
#12470=DIRECTION ( 'NONE',  ( 0.000000000000000000, 0.000000000000000000, -1.000000000000000000 ) ) ;
#12476=VECTOR ( 'NONE', #8835, 1000.000000000000000 ) ;
#12477=CARTESIAN_POINT ( 'NONE',  ( 636.7009106935324780, 155.5114698605638637, -211.0000000000000000 ) ) ;
#12478=VECTOR ( 'NONE', #4250, 1000.000000000000000 ) ;
#12494=DIRECTION ( 'NONE',  ( -0.000000000000000000, -0.000000000000000000, -1.000000000000000000 ) ) ;
#12495=EDGE_CURVE ( 'NONE', #7242, #3214, #7476, .T. ) ;
#12497=FACE_OUTER_BOUND ( 'NONE', #2815, .T. ) ;
#12507=LINE ( 'NONE', #3509, #1911 ) ;
#12524=EDGE_CURVE ( 'NONE', #12114, #11816, #5388, .T. ) ;
#12538=DIRECTION ( 'NONE',  ( -3.469446951953611033E-15, -1.000000000000000000, 0.000000000000000000 ) ) ;
#12554=LINE ( 'NONE', #11507, #14137 ) ;
#12566=CARTESIAN_POINT ( 'NONE',  ( 639.0000000000000000, 156.0000000000000000, -233.5000000000000000 ) ) ;
#12581=EDGE_CURVE ( 'NONE', #9710, #11130, #8447, .T. ) ;
#12584=ORIENTED_EDGE ( 'NONE', *, *, #9413, .T. ) ;
#12600=FACE_OUTER_BOUND ( 'NONE', #1431, .T. ) ;
#12602=EDGE_CURVE ( 'NONE', #5031, #12986, #12208, .T. ) ;
#12603=CARTESIAN_POINT ( 'NONE',  ( 639.0000000000000000, 156.0000000000000000, -233.5000000000000000 ) ) ;
#12663=DIRECTION ( 'NONE',  ( -1.000000000000000000, 0.000000000000000000, 0.000000000000000000 ) ) ;
#12680=ADVANCED_FACE ( 'NONE', ( #14554 ), #5164, .F. ) ;
#12686=EDGE_CURVE ( 'NONE', #3660, #12301, #13529, .T. ) ;
#12695=VECTOR ( 'NONE', #3874, 1000.000000000000227 ) ;
#12698=ORIENTED_EDGE ( 'NONE', *, *, #2474, .F. ) ;
#12743=PRESENTATION_STYLE_ASSIGNMENT (( #10522 ) ) ;
#12768=ORIENTED_EDGE ( 'NONE', *, *, #4137, .F. ) ;
#12786=ORIENTED_EDGE ( 'NONE', *, *, #13968, .F. ) ;
#12788=DIRECTION ( 'NONE',  ( -0.000000000000000000, -0.000000000000000000, 1.000000000000000000 ) ) ;
#12804=DIRECTION ( 'NONE',  ( 0.000000000000000000, 0.000000000000000000, -1.000000000000000000 ) ) ;
#12809=ORIENTED_EDGE ( 'NONE', *, *, #1602, .F. ) ;
#12820=ORIENTED_EDGE ( 'NONE', *, *, #8181, .F. ) ;
#12822=CARTESIAN_POINT ( 'NONE',  ( 636.7717819724297215, 155.3244477714206653, -211.0000000000000000 ) ) ;
#12856=ORIENTED_EDGE ( 'NONE', *, *, #12495, .T. ) ;
#12858=DIRECTION ( 'NONE',  ( -1.000000000000000000, 0.000000000000000000, 0.000000000000000000 ) ) ;
#12861=EDGE_CURVE ( 'NONE', #2242, #9111, #3045, .T. ) ;
#12862=DIRECTION ( 'NONE',  ( -0.000000000000000000, -0.000000000000000000, 1.000000000000000000 ) ) ;
#12894=LINE ( 'NONE', #6107, #10105 ) ;
#12906=VECTOR ( 'NONE', #579, 1000.000000000000000 ) ;
#12911=ORIENTED_EDGE ( 'NONE', *, *, #10247, .T. ) ;
#12932=AXIS2_PLACEMENT_3D ( 'NONE', #2483, #9129, #9354 ) ;
#12942=CARTESIAN_POINT ( 'NONE',  ( 639.0000000000000000, 156.0000000000000000, -225.5000000000000000 ) ) ;
#12951=AXIS2_PLACEMENT_3D ( 'NONE', #8154, #3612, #12663 ) ;
#12955=CARTESIAN_POINT ( 'NONE',  ( 631.0000000000000000, 155.9999999999999432, -233.5000000000000000 ) ) ;
#12962=CARTESIAN_POINT ( 'NONE',  ( 637.0568832135862749, 155.4426727739092655, 211.0000000000000000 ) ) ;
#12973=PLANE ( 'NONE',  #7578 ) ;
#12983=DIRECTION ( 'NONE',  ( -0.000000000000000000, -0.000000000000000000, -1.000000000000000000 ) ) ;
#12986=VERTEX_POINT ( 'NONE', #6781 ) ;
#12987=VECTOR ( 'NONE', #10769, 1000.000000000000000 ) ;
#13019=DIRECTION ( 'NONE',  ( -0.000000000000000000, -0.000000000000000000, -1.000000000000000000 ) ) ;
#13032=ORIENTED_EDGE ( 'NONE', *, *, #2151, .F. ) ;
#13035=CARTESIAN_POINT ( 'NONE',  ( 639.0000000000000000, 156.0000000000000000, -233.5000000000000000 ) ) ;
#13038=PRODUCT ( 'hub', 'hub', '', ( #9971 ) ) ;
#13088=EDGE_CURVE ( 'NONE', #11698, #1513, #10683, .T. ) ;
#13108=CARTESIAN_POINT ( 'NONE',  ( 642.5000000000001137, 160.0000000000000284, -225.5000000000000000 ) ) ;
#13140=EDGE_CURVE ( 'NONE', #10347, #5692, #2496, .T. ) ;
#13142=DIRECTION ( 'NONE',  ( 0.000000000000000000, 0.000000000000000000, -1.000000000000000000 ) ) ;
#13155=VECTOR ( 'NONE', #6004, 1000.000000000000000 ) ;
#13169=AXIS2_PLACEMENT_3D ( 'NONE', #10880, #8656, #2071 ) ;
#13171=LINE ( 'NONE', #3063, #8974 ) ;
#13188=VECTOR ( 'NONE', #2251, 999.9999999999998863 ) ;
#13226=ADVANCED_FACE ( 'NONE', ( #12071 ), #5357, .T. ) ;
#13228=VECTOR ( 'NONE', #12470, 1000.000000000000000 ) ;
#13251=EDGE_CURVE ( 'NONE', #7242, #13261, #6151, .T. ) ;
#13261=VERTEX_POINT ( 'NONE', #8355 ) ;
#13266=EDGE_LOOP ( 'NONE', ( #3551, #5560, #3134, #9957 ) ) ;
#13273=ADVANCED_FACE ( 'NONE', ( #9768 ), #1721, .T. ) ;
#13302=CARTESIAN_POINT ( 'NONE',  ( 635.0000000000000000, 160.0000000000000284, -222.5000000000000000 ) ) ;
#13324=ADVANCED_FACE ( 'NONE', ( #7404 ), #13984, .T. ) ;
#13329=ORIENTED_EDGE ( 'NONE', *, *, #6048, .T. ) ;
#13348=DIRECTION ( 'NONE',  ( 0.000000000000000000, 0.000000000000000000, 1.000000000000000000 ) ) ;
#13359=CIRCLE ( 'NONE', #623, 4.799999999999968736 ) ;
#13387=LINE ( 'NONE', #14503, #1106 ) ;
#13394=AXIS2_PLACEMENT_3D ( 'NONE', #13302, #12180, #8943 ) ;
#13395=VERTEX_POINT ( 'NONE', #2033 ) ;
#13403=AXIS2_PLACEMENT_3D ( 'NONE', #4445, #8944, #7853 ) ;
#13406=CARTESIAN_POINT ( 'NONE',  ( 635.0000000000000000, 160.0000000000000284, -187.5000000000000000 ) ) ;
#13408=DIRECTION ( 'NONE',  ( -1.000000000000000000, 0.000000000000000000, 0.000000000000000000 ) ) ;
#13438=CARTESIAN_POINT ( 'NONE',  ( 635.0000000000000000, 160.0000000000000284, -211.0000000000000000 ) ) ;
#13452=AXIS2_PLACEMENT_3D ( 'NONE', #4580, #12538, #9071 ) ;
#13471=DIRECTION ( 'NONE',  ( 0.000000000000000000, 0.000000000000000000, 1.000000000000000000 ) ) ;
#13477=LINE ( 'NONE', #14, #13678 ) ;
#13500=CARTESIAN_POINT ( 'NONE',  ( 640.0000000000000000, 160.0000000000000284, -222.5000000000000000 ) ) ;
#13519=ORIENTED_EDGE ( 'NONE', *, *, #7454, .F. ) ;
#13527=EDGE_CURVE ( 'NONE', #13261, #3214, #6594, .T. ) ;
#13529=LINE ( 'NONE', #3416, #7027 ) ;
#13531=FACE_BOUND ( 'NONE', #309, .T. ) ;
#13541=CARTESIAN_POINT ( 'NONE',  ( 636.7717819724297215, 155.3244477714206653, 215.5000000000000000 ) ) ;
#13544=CYLINDRICAL_SURFACE ( 'NONE', #11618, 5.000000000000004441 ) ;
#13597=DIRECTION ( 'NONE',  ( 0.000000000000000000, 0.000000000000000000, -1.000000000000000000 ) ) ;
#13602=EDGE_CURVE ( 'NONE', #4648, #4012, #1867, .T. ) ;
#13635=CARTESIAN_POINT ( 'NONE',  ( 635.0000000000000000, 160.0000000000000284, -222.5000000000000000 ) ) ;
#13637=DIRECTION ( 'NONE',  ( 1.000000000000000000, 0.000000000000000000, 0.000000000000000000 ) ) ;
#13642=FACE_OUTER_BOUND ( 'NONE', #7431, .T. ) ;
#13669=VECTOR ( 'NONE', #492, 1000.000000000000000 ) ;
#13672=ORIENTED_EDGE ( 'NONE', *, *, #4228, .T. ) ;
#13678=VECTOR ( 'NONE', #6823, 1000.000000000000000 ) ;
#13681=VECTOR ( 'NONE', #6830, 1000.000000000000000 ) ;
#13687=LINE ( 'NONE', #6965, #1831 ) ;
#13700=EDGE_CURVE ( 'NONE', #7367, #14073, #7881, .T. ) ;
#13705=CARTESIAN_POINT ( 'NONE',  ( 639.0000000000000000, 164.0000000000000000, -233.5000000000000000 ) ) ;
#13717=CIRCLE ( 'NONE', #2403, 5.000000000000004441 ) ;
#13738=EDGE_LOOP ( 'NONE', ( #1399, #867, #12235, #11015, #1112, #7931, #4761, #9177, #3934, #14372, #2935, #8204 ) ) ;
#13740=AXIS2_PLACEMENT_3D ( 'NONE', #6416, #716, #13408 ) ;
#13742=DIRECTION ( 'NONE',  ( -1.000000000000000000, -6.938893903907222067E-15, 0.000000000000000000 ) ) ;
#13787=ORIENTED_EDGE ( 'NONE', *, *, #13527, .F. ) ;
#13791=CARTESIAN_POINT ( 'NONE',  ( 636.9746078850427011, 155.6249658629529620, -210.0000000000000000 ) ) ;
#13817=VERTEX_POINT ( 'NONE', #10519 ) ;
#13837=CIRCLE ( 'NONE', #9836, 4.799999999999968736 ) ;
#13846=( LENGTH_UNIT ( ) NAMED_UNIT ( * ) SI_UNIT ( .MILLI., .METRE. ) );
#13854=PLANE ( 'NONE',  #12932 ) ;
#13856=LINE ( 'NONE', #7950, #13906 ) ;
#13858=( GEOMETRIC_REPRESENTATION_CONTEXT ( 3 ) GLOBAL_UNCERTAINTY_ASSIGNED_CONTEXT ( ( #10942 ) ) GLOBAL_UNIT_ASSIGNED_CONTEXT ( ( #4299, #5541, #4519 ) ) REPRESENTATION_CONTEXT ( 'NONE', 'WORKASPACE' ) );
#13862=EDGE_CURVE ( 'NONE', #9723, #3660, #905, .T. ) ;
#13866=EDGE_LOOP ( 'NONE', ( #9034, #4588, #2995, #4099 ) ) ;
#13886=CARTESIAN_POINT ( 'NONE',  ( 641.0000000000000000, 166.0000000000000284, 187.5000000000000000 ) ) ;
#13896=DIRECTION ( 'NONE',  ( 0.000000000000000000, 0.000000000000000000, -1.000000000000000000 ) ) ;
#13906=VECTOR ( 'NONE', #6850, 1000.000000000000000 ) ;
#13958=ORIENTED_EDGE ( 'NONE', *, *, #14296, .T. ) ;
#13968=EDGE_CURVE ( 'NONE', #5128, #5031, #10607, .T. ) ;
#13984=CYLINDRICAL_SURFACE ( 'NONE', #3530, 5.000000000000004441 ) ;
#14005=CARTESIAN_POINT ( 'NONE',  ( 636.7009106935324780, 155.5114698605638637, -211.0000000000000000 ) ) ;
#14020=CARTESIAN_POINT ( 'NONE',  ( 629.0000000000000000, 154.0000000000000284, -187.5000000000000000 ) ) ;
#14021=DIRECTION ( 'NONE',  ( -0.9237280213470676626, -0.3830490080632388272, 0.000000000000000000 ) ) ;
#14029=ORIENTED_EDGE ( 'NONE', *, *, #13251, .F. ) ;
#14048=EDGE_CURVE ( 'NONE', #2721, #5147, #7992, .T. ) ;
#14073=VERTEX_POINT ( 'NONE', #11178 ) ;
#14100=DIRECTION ( 'NONE',  ( -0.9237280213470676626, -0.3830490080632388272, 0.000000000000000000 ) ) ;
#14101=ORIENTED_EDGE ( 'NONE', *, *, #11799, .F. ) ;
#14109=ORIENTED_EDGE ( 'NONE', *, *, #9512, .T. ) ;
#14120=CARTESIAN_POINT ( 'NONE',  ( 639.4338945024659324, 161.8386352387035743, -210.0000000000000000 ) ) ;
#14133=AXIS2_PLACEMENT_3D ( 'NONE', #6537, #4398, #778 ) ;
#14137=VECTOR ( 'NONE', #2443, 1000.000000000000000 ) ;
#14162=CARTESIAN_POINT ( 'NONE',  ( 629.0000000000000000, 166.0000000000000284, 187.5000000000000000 ) ) ;
#14194=DIRECTION ( 'NONE',  ( 0.000000000000000000, 0.000000000000000000, -1.000000000000000000 ) ) ;
#14199=VECTOR ( 'NONE', #8322, 1000.000000000000000 ) ;
#14212=DIRECTION ( 'NONE',  ( 0.000000000000000000, 0.000000000000000000, -1.000000000000000000 ) ) ;
#14229=DIRECTION ( 'NONE',  ( 1.000000000000000000, 0.000000000000000000, 0.000000000000000000 ) ) ;
#14235=FACE_BOUND ( 'NONE', #7801, .T. ) ;
#14246=LINE ( 'NONE', #4353, #4211 ) ;
#14247=EDGE_CURVE ( 'NONE', #3772, #8326, #4424, .T. ) ;
#14283=ADVANCED_FACE ( 'NONE', ( #7748 ), #669, .T. ) ;
#14292=VERTEX_POINT ( 'NONE', #14120 ) ;
#14296=EDGE_CURVE ( 'NONE', #2721, #12114, #2362, .T. ) ;
#14302=DIRECTION ( 'NONE',  ( 0.000000000000000000, 0.000000000000000000, 1.000000000000000000 ) ) ;
#14306=EDGE_LOOP ( 'NONE', ( #4379, #6839, #12404, #9448 ) ) ;
#14314=LINE ( 'NONE', #8704, #9920 ) ;
#14344=ORIENTED_EDGE ( 'NONE', *, *, #8786, .T. ) ;
#14347=AXIS2_PLACEMENT_3D ( 'NONE', #37, #3678, #8239 ) ;
#14354=ORIENTED_EDGE ( 'NONE', *, *, #8786, .F. ) ;
#14372=ORIENTED_EDGE ( 'NONE', *, *, #12305, .T. ) ;
#14384=AXIS2_PLACEMENT_3D ( 'NONE', #7539, #4300, #5182 ) ;
#14415=ADVANCED_FACE ( 'NONE', ( #10401, #13642 ), #7958, .T. ) ;
#14458=ORIENTED_EDGE ( 'NONE', *, *, #4871, .T. ) ;
#14464=CARTESIAN_POINT ( 'NONE',  ( 627.5000000000000000, 160.0000000000000284, -225.5000000000000000 ) ) ;
#14487=CARTESIAN_POINT ( 'NONE',  ( 635.0000000000000000, 160.0000000000000284, 210.0000000000000000 ) ) ;
#14497=EDGE_CURVE ( 'NONE', #2298, #4638, #5440, .T. ) ;
#14503=CARTESIAN_POINT ( 'NONE',  ( 630.5661054975340676, 158.1613647612965110, 211.0000000000000000 ) ) ;
#14513=ADVANCED_FACE ( 'NONE', ( #10318 ), #2491, .F. ) ;
#14529=ADVANCED_FACE ( 'NONE', ( #11492 ), #2431, .T. ) ;
#14534=DIRECTION ( 'NONE',  ( 0.000000000000000000, 0.000000000000000000, -1.000000000000000000 ) ) ;
#14536=CARTESIAN_POINT ( 'NONE',  ( 631.0000000000000000, 155.9999999999999432, -233.5000000000000000 ) ) ;
#14554=FACE_OUTER_BOUND ( 'NONE', #3839, .T. ) ;
#14557=LINE ( 'NONE', #12477, #5444 ) ;
#14563=AXIS2_PLACEMENT_3D ( 'NONE', #6279, #659, #11950 ) ;
#14570=PLANE ( 'NONE',  #8182 ) ;
#14579=CARTESIAN_POINT ( 'NONE',  ( 635.0000000000000000, 160.0000000000000284, -211.0000000000000000 ) ) ;
#14603=FACE_OUTER_BOUND ( 'NONE', #2656, .T. ) ;
#14615=APPLICATION_CONTEXT ( 'automotive_design' ) ;
#14682=COLOUR_RGB('Off White',0.89,0.88,0.83);
#14683=FILL_AREA_STYLE_COLOUR('',#14682);
#14684=FILL_AREA_STYLE('',(#14683));
#14685=SURFACE_STYLE_FILL_AREA(#14684);
#14686=SURFACE_SIDE_STYLE('',(#14685));
#14687=SURFACE_STYLE_USAGE(.BOTH.,#14686);
#14688=PRESENTATION_STYLE_ASSIGNMENT((#14687));
ENDSEC;
END-ISO-10303-21;
